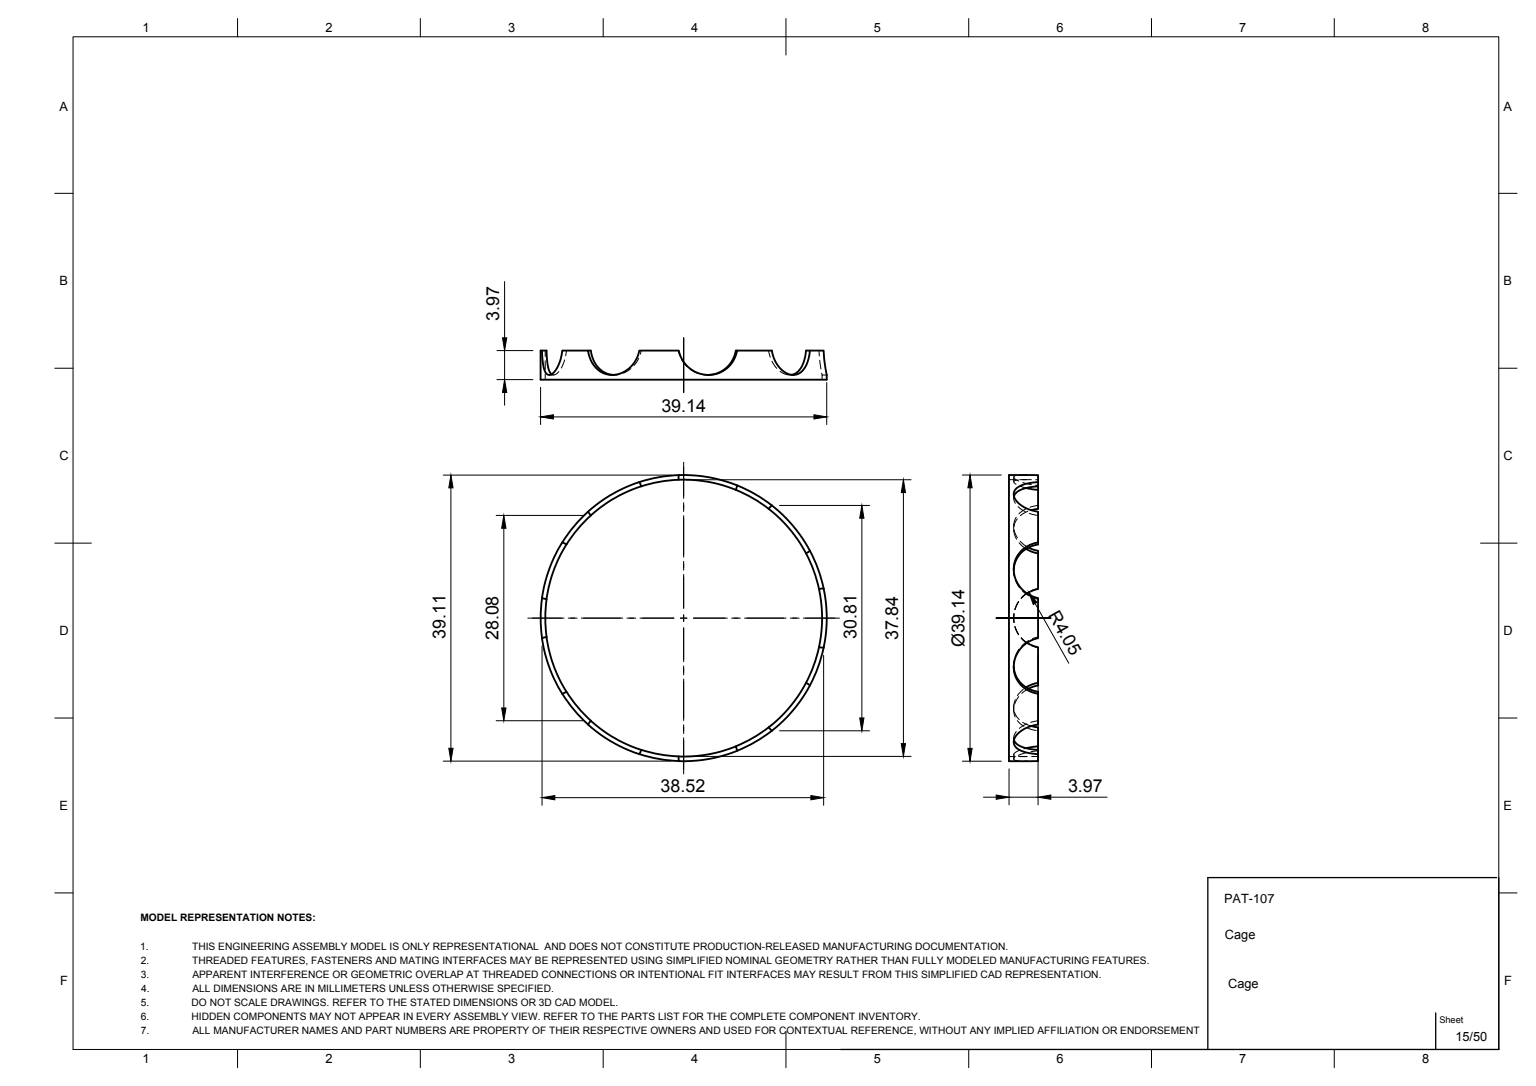
ISO-10303-21;
HEADER;
/* Generated by software containing ST-Developer
 * from STEP Tools, Inc. (www.steptools.com) 
 */

FILE_DESCRIPTION(
/* description */ ('Turntable on roller ring'),
/* implementation_level */ '2;1');

FILE_NAME(
/* name */ 'Cage.step',
/* time_stamp */ '2026-10-28T03:23:59-07:00',
/* author */ (''),
/* organization */ (''),
/* preprocessor_version */ 'ST-DEVELOPER v20.2',
/* originating_system */ 'Autodesk Translation Framework v15.17.0.0',
/* authorisation */ '');

FILE_SCHEMA (('AUTOMOTIVE_DESIGN { 1 0 10303 214 3 1 1 }'));
ENDSEC;

DATA;
#10=MECHANICAL_DESIGN_GEOMETRIC_PRESENTATION_REPRESENTATION('',(#632),#16281);
#399=B_SPLINE_CURVE_WITH_KNOTS('',3,(#13508,#13509,#13510,#13511,#13512,
#13513,#13514,#13515,#13516,#13517,#13518,#13519,#13520,#13521,#13522,#13523,
#13524,#13525,#13526,#13527,#13528,#13529),.UNSPECIFIED.,.F.,.F.,(4,2,2,
2,2,2,2,2,2,2,4),(0.0789043916784349,0.21052649634152,0.31578974451228,
0.421052992683041,0.522171766675512,0.623290540667983,0.724409314660453,
0.825528088652924,0.930791336823684,1.03605458499444,1.16767668965753),
 .UNSPECIFIED.);
#400=B_SPLINE_CURVE_WITH_KNOTS('',3,(#13533,#13534,#13535,#13536,#13537,
#13538,#13539,#13540,#13541,#13542,#13543,#13544,#13545,#13546,#13547,#13548,
#13549,#13550,#13551,#13552,#13553,#13554),.UNSPECIFIED.,.F.,.F.,(4,2,2,
2,2,2,2,2,2,2,4),(0.0774711646211702,0.142095081356994,0.284190162713987,
0.410912155766437,0.514012992401139,0.617113829035841,0.720214665670543,
0.823315502305246,0.950037495357694,1.09213257671469,1.15675649345051),
 .UNSPECIFIED.);
#401=B_SPLINE_CURVE_WITH_KNOTS('',3,(#13560,#13561,#13562,#13563,#13564,
#13565,#13566,#13567,#13568,#13569,#13570,#13571,#13572,#13573,#13574,#13575,
#13576,#13577,#13578,#13579,#13580,#13581),.UNSPECIFIED.,.F.,.F.,(4,2,2,
2,2,2,2,2,2,2,4),(0.0774711646211703,0.142095081356994,0.284190162713988,
0.410912155766436,0.514012992401139,0.617113829035841,0.720214665670544,
0.823315502305246,0.950037495357695,1.09213257671469,1.15675649345051),
 .UNSPECIFIED.);
#402=B_SPLINE_CURVE_WITH_KNOTS('',3,(#13585,#13586,#13587,#13588,#13589,
#13590,#13591,#13592,#13593,#13594,#13595,#13596,#13597,#13598,#13599,#13600,
#13601,#13602,#13603,#13604,#13605,#13606),.UNSPECIFIED.,.F.,.F.,(4,2,2,
2,2,2,2,2,2,2,4),(0.0774711646211702,0.142095081356994,0.284190162713988,
0.410912155766436,0.514012992401139,0.617113829035841,0.720214665670544,
0.823315502305246,0.950037495357695,1.09213257671469,1.15675649345051),
 .UNSPECIFIED.);
#403=B_SPLINE_CURVE_WITH_KNOTS('',3,(#13610,#13611,#13612,#13613,#13614,
#13615,#13616,#13617,#13618,#13619,#13620,#13621,#13622,#13623,#13624,#13625,
#13626,#13627,#13628,#13629,#13630,#13631),.UNSPECIFIED.,.F.,.F.,(4,2,2,
2,2,2,2,2,2,2,4),(0.0774711646211702,0.142095081356994,0.284190162713988,
0.410912155766436,0.514012992401139,0.617113829035842,0.720214665670544,
0.823315502305246,0.950037495357696,1.09213257671469,1.15675649345051),
 .UNSPECIFIED.);
#404=B_SPLINE_CURVE_WITH_KNOTS('',3,(#13640,#13641,#13642,#13643,#13644,
#13645,#13646,#13647,#13648,#13649,#13650,#13651,#13652,#13653,#13654,#13655,
#13656,#13657,#13658,#13659,#13660,#13661),.UNSPECIFIED.,.F.,.F.,(4,2,2,
2,2,2,2,2,2,2,4),(0.0774711646211702,0.142095081356994,0.284190162713987,
0.410912155766436,0.514012992401139,0.617113829035841,0.720214665670543,
0.823315502305246,0.950037495357695,1.09213257671469,1.15675649345051),
 .UNSPECIFIED.);
#405=B_SPLINE_CURVE_WITH_KNOTS('',3,(#13665,#13666,#13667,#13668,#13669,
#13670,#13671,#13672,#13673,#13674,#13675,#13676,#13677,#13678,#13679,#13680,
#13681,#13682,#13683,#13684,#13685,#13686),.UNSPECIFIED.,.F.,.F.,(4,2,2,
2,2,2,2,2,2,2,4),(0.0774711646211702,0.142095081356994,0.284190162713987,
0.410912155766436,0.514012992401139,0.617113829035841,0.720214665670543,
0.823315502305246,0.950037495357695,1.09213257671469,1.15675649345051),
 .UNSPECIFIED.);
#406=B_SPLINE_CURVE_WITH_KNOTS('',3,(#13690,#13691,#13692,#13693,#13694,
#13695,#13696,#13697,#13698,#13699,#13700,#13701,#13702,#13703,#13704,#13705,
#13706,#13707,#13708,#13709,#13710,#13711),.UNSPECIFIED.,.F.,.F.,(4,2,2,
2,2,2,2,2,2,2,4),(0.0774711646211703,0.142095081356994,0.284190162713988,
0.410912155766437,0.514012992401139,0.617113829035841,0.720214665670544,
0.823315502305247,0.950037495357696,1.09213257671469,1.15675649345051),
 .UNSPECIFIED.);
#407=B_SPLINE_CURVE_WITH_KNOTS('',3,(#13715,#13716,#13717,#13718,#13719,
#13720,#13721,#13722,#13723,#13724,#13725,#13726,#13727,#13728,#13729,#13730,
#13731,#13732,#13733,#13734,#13735,#13736),.UNSPECIFIED.,.F.,.F.,(4,2,2,
2,2,2,2,2,2,2,4),(0.0774711646211703,0.142095081356994,0.284190162713987,
0.410912155766436,0.514012992401139,0.617113829035841,0.720214665670543,
0.823315502305245,0.950037495357694,1.09213257671469,1.15675649345051),
 .UNSPECIFIED.);
#408=B_SPLINE_CURVE_WITH_KNOTS('',3,(#13740,#13741,#13742,#13743,#13744,
#13745,#13746,#13747,#13748,#13749,#13750,#13751,#13752,#13753,#13754,#13755,
#13756,#13757,#13758,#13759,#13760,#13761),.UNSPECIFIED.,.F.,.F.,(4,2,2,
2,2,2,2,2,2,2,4),(0.0774711646211703,0.142095081356994,0.284190162713988,
0.410912155766437,0.514012992401139,0.617113829035841,0.720214665670544,
0.823315502305246,0.950037495357695,1.09213257671469,1.15675649345051),
 .UNSPECIFIED.);
#409=B_SPLINE_CURVE_WITH_KNOTS('',3,(#13769,#13770,#13771,#13772,#13773,
#13774,#13775,#13776,#13777,#13778,#13779,#13780,#13781,#13782,#13783,#13784,
#13785,#13786,#13787,#13788,#13789,#13790),.UNSPECIFIED.,.F.,.F.,(4,2,2,
2,2,2,2,2,2,2,4),(0.0789043916784349,0.21052649634152,0.315789744512281,
0.421052992683041,0.522171766675512,0.623290540667983,0.724409314660453,
0.825528088652924,0.930791336823684,1.03605458499444,1.16767668965753),
 .UNSPECIFIED.);
#410=B_SPLINE_CURVE_WITH_KNOTS('',3,(#13798,#13799,#13800,#13801,#13802,
#13803,#13804,#13805,#13806,#13807,#13808,#13809,#13810,#13811,#13812,#13813,
#13814,#13815,#13816,#13817,#13818,#13819),.UNSPECIFIED.,.F.,.F.,(4,2,2,
2,2,2,2,2,2,2,4),(0.0789043916784348,0.210526496341521,0.315789744512281,
0.421052992683042,0.522171766675513,0.623290540667983,0.724409314660454,
0.825528088652925,0.930791336823685,1.03605458499444,1.16767668965753),
 .UNSPECIFIED.);
#411=B_SPLINE_CURVE_WITH_KNOTS('',3,(#13827,#13828,#13829,#13830,#13831,
#13832,#13833,#13834,#13835,#13836,#13837,#13838,#13839,#13840,#13841,#13842,
#13843,#13844,#13845,#13846,#13847,#13848),.UNSPECIFIED.,.F.,.F.,(4,2,2,
2,2,2,2,2,2,2,4),(0.0789043916784349,0.21052649634152,0.31578974451228,
0.421052992683041,0.522171766675511,0.623290540667982,0.724409314660453,
0.825528088652924,0.930791336823685,1.03605458499444,1.16767668965753),
 .UNSPECIFIED.);
#412=B_SPLINE_CURVE_WITH_KNOTS('',3,(#13858,#13859,#13860,#13861,#13862,
#13863,#13864,#13865,#13866,#13867,#13868,#13869,#13870,#13871,#13872,#13873,
#13874,#13875,#13876,#13877,#13878,#13879),.UNSPECIFIED.,.F.,.F.,(4,2,2,
2,2,2,2,2,2,2,4),(0.0789043916784348,0.21052649634152,0.315789744512281,
0.421052992683041,0.522171766675511,0.623290540667982,0.724409314660453,
0.825528088652924,0.930791336823684,1.03605458499444,1.16767668965753),
 .UNSPECIFIED.);
#413=B_SPLINE_CURVE_WITH_KNOTS('',3,(#13887,#13888,#13889,#13890,#13891,
#13892,#13893,#13894,#13895,#13896,#13897,#13898,#13899,#13900,#13901,#13902,
#13903,#13904,#13905,#13906,#13907,#13908),.UNSPECIFIED.,.F.,.F.,(4,2,2,
2,2,2,2,2,2,2,4),(0.0789043916784348,0.21052649634152,0.31578974451228,
0.42105299268304,0.522171766675511,0.623290540667982,0.724409314660453,
0.825528088652924,0.930791336823684,1.03605458499444,1.16767668965753),
 .UNSPECIFIED.);
#414=B_SPLINE_CURVE_WITH_KNOTS('',3,(#13916,#13917,#13918,#13919,#13920,
#13921,#13922,#13923,#13924,#13925,#13926,#13927,#13928,#13929,#13930,#13931,
#13932,#13933,#13934,#13935,#13936,#13937),.UNSPECIFIED.,.F.,.F.,(4,2,2,
2,2,2,2,2,2,2,4),(0.0789043916784348,0.21052649634152,0.315789744512281,
0.421052992683041,0.522171766675512,0.623290540667982,0.724409314660453,
0.825528088652924,0.930791336823684,1.03605458499444,1.16767668965753),
 .UNSPECIFIED.);
#415=B_SPLINE_CURVE_WITH_KNOTS('',3,(#13945,#13946,#13947,#13948,#13949,
#13950,#13951,#13952,#13953,#13954,#13955,#13956,#13957,#13958,#13959,#13960,
#13961,#13962,#13963,#13964,#13965,#13966),.UNSPECIFIED.,.F.,.F.,(4,2,2,
2,2,2,2,2,2,2,4),(0.0789043916784349,0.21052649634152,0.31578974451228,
0.42105299268304,0.522171766675511,0.623290540667982,0.724409314660453,
0.825528088652924,0.930791336823684,1.03605458499444,1.16767668965753),
 .UNSPECIFIED.);
#416=B_SPLINE_CURVE_WITH_KNOTS('',3,(#13975,#13976,#13977,#13978,#13979,
#13980,#13981,#13982,#13983,#13984,#13985,#13986,#13987,#13988,#13989,#13990,
#13991,#13992,#13993,#13994,#13995,#13996),.UNSPECIFIED.,.F.,.F.,(4,2,2,
2,2,2,2,2,2,2,4),(0.0789043916784348,0.21052649634152,0.31578974451228,
0.42105299268304,0.522171766675511,0.623290540667982,0.724409314660453,
0.825528088652924,0.930791336823684,1.03605458499444,1.16767668965753),
 .UNSPECIFIED.);
#447=SPHERICAL_SURFACE('',#9291,0.412776);
#448=SPHERICAL_SURFACE('',#9309,0.412776);
#449=SPHERICAL_SURFACE('',#9314,0.412776);
#450=SPHERICAL_SURFACE('',#9319,0.412776);
#451=SPHERICAL_SURFACE('',#9325,0.412776);
#452=SPHERICAL_SURFACE('',#9330,0.412776);
#453=SPHERICAL_SURFACE('',#9335,0.412776);
#454=SPHERICAL_SURFACE('',#9340,0.412776);
#455=SPHERICAL_SURFACE('',#9348,0.412776);
#514=SHAPE_REPRESENTATION_RELATIONSHIP('SRR','None',#16529,#569);
#569=ADVANCED_BREP_SHAPE_REPRESENTATION('',(#703),#16223);
#632=STYLED_ITEM('',(#16932),#703);
#703=MANIFOLD_SOLID_BREP('Continuous crown cage',#8374);
#828=FACE_BOUND('',#1953,.T.);
#1025=PLANE('',#9306);
#1026=PLANE('',#9311);
#1027=PLANE('',#9316);
#1028=PLANE('',#9321);
#1029=PLANE('',#9327);
#1030=PLANE('',#9332);
#1031=PLANE('',#9337);
#1032=PLANE('',#9346);
#1033=PLANE('',#9350);
#1034=PLANE('',#9351);
#1357=FACE_OUTER_BOUND('',#1933,.T.);
#1358=FACE_OUTER_BOUND('',#1934,.T.);
#1359=FACE_OUTER_BOUND('',#1935,.T.);
#1360=FACE_OUTER_BOUND('',#1936,.T.);
#1361=FACE_OUTER_BOUND('',#1937,.T.);
#1362=FACE_OUTER_BOUND('',#1938,.T.);
#1363=FACE_OUTER_BOUND('',#1939,.T.);
#1364=FACE_OUTER_BOUND('',#1940,.T.);
#1365=FACE_OUTER_BOUND('',#1941,.T.);
#1366=FACE_OUTER_BOUND('',#1942,.T.);
#1367=FACE_OUTER_BOUND('',#1943,.T.);
#1368=FACE_OUTER_BOUND('',#1944,.T.);
#1369=FACE_OUTER_BOUND('',#1945,.T.);
#1370=FACE_OUTER_BOUND('',#1946,.T.);
#1371=FACE_OUTER_BOUND('',#1947,.T.);
#1372=FACE_OUTER_BOUND('',#1948,.T.);
#1373=FACE_OUTER_BOUND('',#1949,.T.);
#1374=FACE_OUTER_BOUND('',#1950,.T.);
#1375=FACE_OUTER_BOUND('',#1951,.T.);
#1376=FACE_OUTER_BOUND('',#1952,.T.);
#1377=FACE_OUTER_BOUND('',#1954,.T.);
#1933=EDGE_LOOP('',(#6101,#6102,#6103,#6104));
#1934=EDGE_LOOP('',(#6105,#6106,#6107,#6108,#6109,#6110,#6111,#6112,#6113,
#6114,#6115,#6116,#6117,#6118,#6119,#6120,#6121,#6122,#6123,#6124,#6125,
#6126));
#1935=EDGE_LOOP('',(#6127,#6128,#6129,#6130));
#1936=EDGE_LOOP('',(#6131,#6132,#6133,#6134));
#1937=EDGE_LOOP('',(#6135,#6136,#6137,#6138));
#1938=EDGE_LOOP('',(#6139,#6140,#6141,#6142));
#1939=EDGE_LOOP('',(#6143,#6144,#6145,#6146));
#1940=EDGE_LOOP('',(#6147,#6148,#6149,#6150));
#1941=EDGE_LOOP('',(#6151,#6152,#6153,#6154,#6155,#6156));
#1942=EDGE_LOOP('',(#6157,#6158,#6159,#6160));
#1943=EDGE_LOOP('',(#6161,#6162,#6163,#6164));
#1944=EDGE_LOOP('',(#6165,#6166,#6167,#6168));
#1945=EDGE_LOOP('',(#6169,#6170,#6171,#6172));
#1946=EDGE_LOOP('',(#6173,#6174,#6175,#6176));
#1947=EDGE_LOOP('',(#6177,#6178,#6179,#6180));
#1948=EDGE_LOOP('',(#6181,#6182,#6183,#6184));
#1949=EDGE_LOOP('',(#6185,#6186,#6187,#6188,#6189,#6190,#6191,#6192,#6193,
#6194,#6195,#6196,#6197,#6198,#6199,#6200,#6201,#6202,#6203,#6204,#6205,
#6206));
#1950=EDGE_LOOP('',(#6207,#6208,#6209,#6210));
#1951=EDGE_LOOP('',(#6211,#6212,#6213,#6214));
#1952=EDGE_LOOP('',(#6215));
#1953=EDGE_LOOP('',(#6216));
#1954=EDGE_LOOP('',(#6217,#6218,#6219,#6220));
#2588=LINE('',#13635,#3071);
#2589=LINE('',#13971,#3072);
#3071=VECTOR('',#10813,1.956752);
#3072=VECTOR('',#10904,1.893248);
#3592=CIRCLE('',#9292,0.405071403305639);
#3593=CIRCLE('',#9293,0.405071403305639);
#3594=CIRCLE('',#9295,1.956752);
#3595=CIRCLE('',#9296,1.956752);
#3596=CIRCLE('',#9297,1.956752);
#3597=CIRCLE('',#9298,1.956752);
#3598=CIRCLE('',#9299,1.956752);
#3599=CIRCLE('',#9300,1.956752);
#3600=CIRCLE('',#9301,1.956752);
#3601=CIRCLE('',#9302,1.956752);
#3602=CIRCLE('',#9303,1.956752);
#3603=CIRCLE('',#9304,1.956752);
#3604=CIRCLE('',#9305,1.956752);
#3605=CIRCLE('',#9307,1.893248);
#3606=CIRCLE('',#9308,0.405071403305639);
#3607=CIRCLE('',#9310,0.405071403305639);
#3608=CIRCLE('',#9312,1.893248);
#3609=CIRCLE('',#9313,0.405071403305639);
#3610=CIRCLE('',#9315,0.405071403305639);
#3611=CIRCLE('',#9317,1.893248);
#3612=CIRCLE('',#9318,0.405071403305639);
#3613=CIRCLE('',#9320,0.405071403305639);
#3614=CIRCLE('',#9322,1.893248);
#3615=CIRCLE('',#9323,1.893248);
#3616=CIRCLE('',#9324,0.405071403305639);
#3617=CIRCLE('',#9326,0.405071403305639);
#3618=CIRCLE('',#9328,1.893248);
#3619=CIRCLE('',#9329,0.405071403305639);
#3620=CIRCLE('',#9331,0.405071403305639);
#3621=CIRCLE('',#9333,1.893248);
#3622=CIRCLE('',#9334,0.405071403305639);
#3623=CIRCLE('',#9336,0.405071403305639);
#3624=CIRCLE('',#9338,1.893248);
#3625=CIRCLE('',#9339,0.405071403305639);
#3626=CIRCLE('',#9341,0.405071403305639);
#3627=CIRCLE('',#9343,1.893248);
#3628=CIRCLE('',#9344,1.893248);
#3629=CIRCLE('',#9345,1.893248);
#3630=CIRCLE('',#9347,0.405071403305639);
#3631=CIRCLE('',#9349,0.405071403305639);
#4105=VERTEX_POINT('',#13506);
#4106=VERTEX_POINT('',#13507);
#4107=VERTEX_POINT('',#13530);
#4108=VERTEX_POINT('',#13532);
#4109=VERTEX_POINT('',#13557);
#4110=VERTEX_POINT('',#13559);
#4111=VERTEX_POINT('',#13582);
#4112=VERTEX_POINT('',#13584);
#4113=VERTEX_POINT('',#13607);
#4114=VERTEX_POINT('',#13609);
#4115=VERTEX_POINT('',#13632);
#4116=VERTEX_POINT('',#13634);
#4117=VERTEX_POINT('',#13637);
#4118=VERTEX_POINT('',#13639);
#4119=VERTEX_POINT('',#13662);
#4120=VERTEX_POINT('',#13664);
#4121=VERTEX_POINT('',#13687);
#4122=VERTEX_POINT('',#13689);
#4123=VERTEX_POINT('',#13712);
#4124=VERTEX_POINT('',#13714);
#4125=VERTEX_POINT('',#13737);
#4126=VERTEX_POINT('',#13739);
#4127=VERTEX_POINT('',#13764);
#4128=VERTEX_POINT('',#13768);
#4129=VERTEX_POINT('',#13793);
#4130=VERTEX_POINT('',#13797);
#4131=VERTEX_POINT('',#13822);
#4132=VERTEX_POINT('',#13826);
#4133=VERTEX_POINT('',#13851);
#4134=VERTEX_POINT('',#13853);
#4135=VERTEX_POINT('',#13857);
#4136=VERTEX_POINT('',#13882);
#4137=VERTEX_POINT('',#13886);
#4138=VERTEX_POINT('',#13911);
#4139=VERTEX_POINT('',#13915);
#4140=VERTEX_POINT('',#13940);
#4141=VERTEX_POINT('',#13944);
#4142=VERTEX_POINT('',#13969);
#4143=VERTEX_POINT('',#13972);
#4144=VERTEX_POINT('',#13974);
#4861=EDGE_CURVE('',#4105,#4106,#399,.T.);
#4862=EDGE_CURVE('',#4107,#4105,#3592,.T.);
#4863=EDGE_CURVE('',#4108,#4107,#400,.T.);
#4864=EDGE_CURVE('',#4106,#4108,#3593,.T.);
#4865=EDGE_CURVE('',#4109,#4107,#3594,.T.);
#4866=EDGE_CURVE('',#4109,#4110,#401,.T.);
#4867=EDGE_CURVE('',#4111,#4110,#3595,.T.);
#4868=EDGE_CURVE('',#4111,#4112,#402,.T.);
#4869=EDGE_CURVE('',#4113,#4112,#3596,.T.);
#4870=EDGE_CURVE('',#4113,#4114,#403,.T.);
#4871=EDGE_CURVE('',#4115,#4114,#3597,.T.);
#4872=EDGE_CURVE('',#4115,#4116,#2588,.T.);
#4873=EDGE_CURVE('',#4116,#4116,#3598,.T.);
#4874=EDGE_CURVE('',#4117,#4115,#3599,.T.);
#4875=EDGE_CURVE('',#4117,#4118,#404,.T.);
#4876=EDGE_CURVE('',#4119,#4118,#3600,.T.);
#4877=EDGE_CURVE('',#4119,#4120,#405,.T.);
#4878=EDGE_CURVE('',#4121,#4120,#3601,.T.);
#4879=EDGE_CURVE('',#4121,#4122,#406,.T.);
#4880=EDGE_CURVE('',#4123,#4122,#3602,.T.);
#4881=EDGE_CURVE('',#4123,#4124,#407,.T.);
#4882=EDGE_CURVE('',#4125,#4124,#3603,.T.);
#4883=EDGE_CURVE('',#4125,#4126,#408,.T.);
#4884=EDGE_CURVE('',#4108,#4126,#3604,.T.);
#4885=EDGE_CURVE('',#4105,#4127,#3605,.T.);
#4886=EDGE_CURVE('',#4127,#4109,#3606,.T.);
#4887=EDGE_CURVE('',#4128,#4127,#409,.T.);
#4888=EDGE_CURVE('',#4110,#4128,#3607,.T.);
#4889=EDGE_CURVE('',#4128,#4129,#3608,.T.);
#4890=EDGE_CURVE('',#4129,#4111,#3609,.T.);
#4891=EDGE_CURVE('',#4130,#4129,#410,.T.);
#4892=EDGE_CURVE('',#4112,#4130,#3610,.T.);
#4893=EDGE_CURVE('',#4130,#4131,#3611,.T.);
#4894=EDGE_CURVE('',#4131,#4113,#3612,.T.);
#4895=EDGE_CURVE('',#4132,#4131,#411,.T.);
#4896=EDGE_CURVE('',#4114,#4132,#3613,.T.);
#4897=EDGE_CURVE('',#4132,#4133,#3614,.T.);
#4898=EDGE_CURVE('',#4133,#4134,#3615,.T.);
#4899=EDGE_CURVE('',#4134,#4117,#3616,.T.);
#4900=EDGE_CURVE('',#4135,#4134,#412,.T.);
#4901=EDGE_CURVE('',#4118,#4135,#3617,.T.);
#4902=EDGE_CURVE('',#4135,#4136,#3618,.T.);
#4903=EDGE_CURVE('',#4136,#4119,#3619,.T.);
#4904=EDGE_CURVE('',#4137,#4136,#413,.T.);
#4905=EDGE_CURVE('',#4120,#4137,#3620,.T.);
#4906=EDGE_CURVE('',#4137,#4138,#3621,.T.);
#4907=EDGE_CURVE('',#4138,#4121,#3622,.T.);
#4908=EDGE_CURVE('',#4139,#4138,#414,.T.);
#4909=EDGE_CURVE('',#4122,#4139,#3623,.T.);
#4910=EDGE_CURVE('',#4139,#4140,#3624,.T.);
#4911=EDGE_CURVE('',#4140,#4123,#3625,.T.);
#4912=EDGE_CURVE('',#4141,#4140,#415,.T.);
#4913=EDGE_CURVE('',#4124,#4141,#3626,.T.);
#4914=EDGE_CURVE('',#4142,#4142,#3627,.T.);
#4915=EDGE_CURVE('',#4142,#4133,#2589,.T.);
#4916=EDGE_CURVE('',#4143,#4106,#3628,.T.);
#4917=EDGE_CURVE('',#4143,#4144,#416,.T.);
#4918=EDGE_CURVE('',#4141,#4144,#3629,.T.);
#4919=EDGE_CURVE('',#4126,#4143,#3630,.T.);
#4920=EDGE_CURVE('',#4144,#4125,#3631,.T.);
#6101=ORIENTED_EDGE('',*,*,#4861,.F.);
#6102=ORIENTED_EDGE('',*,*,#4862,.F.);
#6103=ORIENTED_EDGE('',*,*,#4863,.F.);
#6104=ORIENTED_EDGE('',*,*,#4864,.F.);
#6105=ORIENTED_EDGE('',*,*,#4863,.T.);
#6106=ORIENTED_EDGE('',*,*,#4865,.F.);
#6107=ORIENTED_EDGE('',*,*,#4866,.T.);
#6108=ORIENTED_EDGE('',*,*,#4867,.F.);
#6109=ORIENTED_EDGE('',*,*,#4868,.T.);
#6110=ORIENTED_EDGE('',*,*,#4869,.F.);
#6111=ORIENTED_EDGE('',*,*,#4870,.T.);
#6112=ORIENTED_EDGE('',*,*,#4871,.F.);
#6113=ORIENTED_EDGE('',*,*,#4872,.T.);
#6114=ORIENTED_EDGE('',*,*,#4873,.F.);
#6115=ORIENTED_EDGE('',*,*,#4872,.F.);
#6116=ORIENTED_EDGE('',*,*,#4874,.F.);
#6117=ORIENTED_EDGE('',*,*,#4875,.T.);
#6118=ORIENTED_EDGE('',*,*,#4876,.F.);
#6119=ORIENTED_EDGE('',*,*,#4877,.T.);
#6120=ORIENTED_EDGE('',*,*,#4878,.F.);
#6121=ORIENTED_EDGE('',*,*,#4879,.T.);
#6122=ORIENTED_EDGE('',*,*,#4880,.F.);
#6123=ORIENTED_EDGE('',*,*,#4881,.T.);
#6124=ORIENTED_EDGE('',*,*,#4882,.F.);
#6125=ORIENTED_EDGE('',*,*,#4883,.T.);
#6126=ORIENTED_EDGE('',*,*,#4884,.F.);
#6127=ORIENTED_EDGE('',*,*,#4862,.T.);
#6128=ORIENTED_EDGE('',*,*,#4885,.T.);
#6129=ORIENTED_EDGE('',*,*,#4886,.T.);
#6130=ORIENTED_EDGE('',*,*,#4865,.T.);
#6131=ORIENTED_EDGE('',*,*,#4887,.F.);
#6132=ORIENTED_EDGE('',*,*,#4888,.F.);
#6133=ORIENTED_EDGE('',*,*,#4866,.F.);
#6134=ORIENTED_EDGE('',*,*,#4886,.F.);
#6135=ORIENTED_EDGE('',*,*,#4888,.T.);
#6136=ORIENTED_EDGE('',*,*,#4889,.T.);
#6137=ORIENTED_EDGE('',*,*,#4890,.T.);
#6138=ORIENTED_EDGE('',*,*,#4867,.T.);
#6139=ORIENTED_EDGE('',*,*,#4891,.F.);
#6140=ORIENTED_EDGE('',*,*,#4892,.F.);
#6141=ORIENTED_EDGE('',*,*,#4868,.F.);
#6142=ORIENTED_EDGE('',*,*,#4890,.F.);
#6143=ORIENTED_EDGE('',*,*,#4892,.T.);
#6144=ORIENTED_EDGE('',*,*,#4893,.T.);
#6145=ORIENTED_EDGE('',*,*,#4894,.T.);
#6146=ORIENTED_EDGE('',*,*,#4869,.T.);
#6147=ORIENTED_EDGE('',*,*,#4895,.F.);
#6148=ORIENTED_EDGE('',*,*,#4896,.F.);
#6149=ORIENTED_EDGE('',*,*,#4870,.F.);
#6150=ORIENTED_EDGE('',*,*,#4894,.F.);
#6151=ORIENTED_EDGE('',*,*,#4896,.T.);
#6152=ORIENTED_EDGE('',*,*,#4897,.T.);
#6153=ORIENTED_EDGE('',*,*,#4898,.T.);
#6154=ORIENTED_EDGE('',*,*,#4899,.T.);
#6155=ORIENTED_EDGE('',*,*,#4874,.T.);
#6156=ORIENTED_EDGE('',*,*,#4871,.T.);
#6157=ORIENTED_EDGE('',*,*,#4900,.F.);
#6158=ORIENTED_EDGE('',*,*,#4901,.F.);
#6159=ORIENTED_EDGE('',*,*,#4875,.F.);
#6160=ORIENTED_EDGE('',*,*,#4899,.F.);
#6161=ORIENTED_EDGE('',*,*,#4901,.T.);
#6162=ORIENTED_EDGE('',*,*,#4902,.T.);
#6163=ORIENTED_EDGE('',*,*,#4903,.T.);
#6164=ORIENTED_EDGE('',*,*,#4876,.T.);
#6165=ORIENTED_EDGE('',*,*,#4904,.F.);
#6166=ORIENTED_EDGE('',*,*,#4905,.F.);
#6167=ORIENTED_EDGE('',*,*,#4877,.F.);
#6168=ORIENTED_EDGE('',*,*,#4903,.F.);
#6169=ORIENTED_EDGE('',*,*,#4905,.T.);
#6170=ORIENTED_EDGE('',*,*,#4906,.T.);
#6171=ORIENTED_EDGE('',*,*,#4907,.T.);
#6172=ORIENTED_EDGE('',*,*,#4878,.T.);
#6173=ORIENTED_EDGE('',*,*,#4908,.F.);
#6174=ORIENTED_EDGE('',*,*,#4909,.F.);
#6175=ORIENTED_EDGE('',*,*,#4879,.F.);
#6176=ORIENTED_EDGE('',*,*,#4907,.F.);
#6177=ORIENTED_EDGE('',*,*,#4909,.T.);
#6178=ORIENTED_EDGE('',*,*,#4910,.T.);
#6179=ORIENTED_EDGE('',*,*,#4911,.T.);
#6180=ORIENTED_EDGE('',*,*,#4880,.T.);
#6181=ORIENTED_EDGE('',*,*,#4881,.F.);
#6182=ORIENTED_EDGE('',*,*,#4911,.F.);
#6183=ORIENTED_EDGE('',*,*,#4912,.F.);
#6184=ORIENTED_EDGE('',*,*,#4913,.F.);
#6185=ORIENTED_EDGE('',*,*,#4914,.F.);
#6186=ORIENTED_EDGE('',*,*,#4915,.T.);
#6187=ORIENTED_EDGE('',*,*,#4897,.F.);
#6188=ORIENTED_EDGE('',*,*,#4895,.T.);
#6189=ORIENTED_EDGE('',*,*,#4893,.F.);
#6190=ORIENTED_EDGE('',*,*,#4891,.T.);
#6191=ORIENTED_EDGE('',*,*,#4889,.F.);
#6192=ORIENTED_EDGE('',*,*,#4887,.T.);
#6193=ORIENTED_EDGE('',*,*,#4885,.F.);
#6194=ORIENTED_EDGE('',*,*,#4861,.T.);
#6195=ORIENTED_EDGE('',*,*,#4916,.F.);
#6196=ORIENTED_EDGE('',*,*,#4917,.T.);
#6197=ORIENTED_EDGE('',*,*,#4918,.F.);
#6198=ORIENTED_EDGE('',*,*,#4912,.T.);
#6199=ORIENTED_EDGE('',*,*,#4910,.F.);
#6200=ORIENTED_EDGE('',*,*,#4908,.T.);
#6201=ORIENTED_EDGE('',*,*,#4906,.F.);
#6202=ORIENTED_EDGE('',*,*,#4904,.T.);
#6203=ORIENTED_EDGE('',*,*,#4902,.F.);
#6204=ORIENTED_EDGE('',*,*,#4900,.T.);
#6205=ORIENTED_EDGE('',*,*,#4898,.F.);
#6206=ORIENTED_EDGE('',*,*,#4915,.F.);
#6207=ORIENTED_EDGE('',*,*,#4864,.T.);
#6208=ORIENTED_EDGE('',*,*,#4884,.T.);
#6209=ORIENTED_EDGE('',*,*,#4919,.T.);
#6210=ORIENTED_EDGE('',*,*,#4916,.T.);
#6211=ORIENTED_EDGE('',*,*,#4883,.F.);
#6212=ORIENTED_EDGE('',*,*,#4920,.F.);
#6213=ORIENTED_EDGE('',*,*,#4917,.F.);
#6214=ORIENTED_EDGE('',*,*,#4919,.F.);
#6215=ORIENTED_EDGE('',*,*,#4873,.T.);
#6216=ORIENTED_EDGE('',*,*,#4914,.T.);
#6217=ORIENTED_EDGE('',*,*,#4913,.T.);
#6218=ORIENTED_EDGE('',*,*,#4918,.T.);
#6219=ORIENTED_EDGE('',*,*,#4920,.T.);
#6220=ORIENTED_EDGE('',*,*,#4882,.T.);
#7723=CYLINDRICAL_SURFACE('',#9294,1.956752);
#7724=CYLINDRICAL_SURFACE('',#9342,1.893248);
#7960=ADVANCED_FACE('',(#1357),#447,.F.);
#7961=ADVANCED_FACE('',(#1358),#7723,.T.);
#7962=ADVANCED_FACE('',(#1359),#1025,.T.);
#7963=ADVANCED_FACE('',(#1360),#448,.F.);
#7964=ADVANCED_FACE('',(#1361),#1026,.T.);
#7965=ADVANCED_FACE('',(#1362),#449,.F.);
#7966=ADVANCED_FACE('',(#1363),#1027,.T.);
#7967=ADVANCED_FACE('',(#1364),#450,.F.);
#7968=ADVANCED_FACE('',(#1365),#1028,.T.);
#7969=ADVANCED_FACE('',(#1366),#451,.F.);
#7970=ADVANCED_FACE('',(#1367),#1029,.T.);
#7971=ADVANCED_FACE('',(#1368),#452,.F.);
#7972=ADVANCED_FACE('',(#1369),#1030,.T.);
#7973=ADVANCED_FACE('',(#1370),#453,.F.);
#7974=ADVANCED_FACE('',(#1371),#1031,.T.);
#7975=ADVANCED_FACE('',(#1372),#454,.F.);
#7976=ADVANCED_FACE('',(#1373),#7724,.F.);
#7977=ADVANCED_FACE('',(#1374),#1032,.T.);
#7978=ADVANCED_FACE('',(#1375),#455,.F.);
#7979=ADVANCED_FACE('',(#1376,#828),#1033,.T.);
#7980=ADVANCED_FACE('',(#1377),#1034,.T.);
#8374=CLOSED_SHELL('',(#7960,#7961,#7962,#7963,#7964,#7965,#7966,#7967,
#7968,#7969,#7970,#7971,#7972,#7973,#7974,#7975,#7976,#7977,#7978,#7979,
#7980));
#9290=AXIS2_PLACEMENT_3D('',#13504,#10795,#10796);
#9291=AXIS2_PLACEMENT_3D('',#13505,#10797,#10798);
#9292=AXIS2_PLACEMENT_3D('',#13531,#10799,#10800);
#9293=AXIS2_PLACEMENT_3D('',#13555,#10801,#10802);
#9294=AXIS2_PLACEMENT_3D('',#13556,#10803,#10804);
#9295=AXIS2_PLACEMENT_3D('',#13558,#10805,#10806);
#9296=AXIS2_PLACEMENT_3D('',#13583,#10807,#10808);
#9297=AXIS2_PLACEMENT_3D('',#13608,#10809,#10810);
#9298=AXIS2_PLACEMENT_3D('',#13633,#10811,#10812);
#9299=AXIS2_PLACEMENT_3D('',#13636,#10814,#10815);
#9300=AXIS2_PLACEMENT_3D('',#13638,#10816,#10817);
#9301=AXIS2_PLACEMENT_3D('',#13663,#10818,#10819);
#9302=AXIS2_PLACEMENT_3D('',#13688,#10820,#10821);
#9303=AXIS2_PLACEMENT_3D('',#13713,#10822,#10823);
#9304=AXIS2_PLACEMENT_3D('',#13738,#10824,#10825);
#9305=AXIS2_PLACEMENT_3D('',#13762,#10826,#10827);
#9306=AXIS2_PLACEMENT_3D('',#13763,#10828,#10829);
#9307=AXIS2_PLACEMENT_3D('',#13765,#10830,#10831);
#9308=AXIS2_PLACEMENT_3D('',#13766,#10832,#10833);
#9309=AXIS2_PLACEMENT_3D('',#13767,#10834,#10835);
#9310=AXIS2_PLACEMENT_3D('',#13791,#10836,#10837);
#9311=AXIS2_PLACEMENT_3D('',#13792,#10838,#10839);
#9312=AXIS2_PLACEMENT_3D('',#13794,#10840,#10841);
#9313=AXIS2_PLACEMENT_3D('',#13795,#10842,#10843);
#9314=AXIS2_PLACEMENT_3D('',#13796,#10844,#10845);
#9315=AXIS2_PLACEMENT_3D('',#13820,#10846,#10847);
#9316=AXIS2_PLACEMENT_3D('',#13821,#10848,#10849);
#9317=AXIS2_PLACEMENT_3D('',#13823,#10850,#10851);
#9318=AXIS2_PLACEMENT_3D('',#13824,#10852,#10853);
#9319=AXIS2_PLACEMENT_3D('',#13825,#10854,#10855);
#9320=AXIS2_PLACEMENT_3D('',#13849,#10856,#10857);
#9321=AXIS2_PLACEMENT_3D('',#13850,#10858,#10859);
#9322=AXIS2_PLACEMENT_3D('',#13852,#10860,#10861);
#9323=AXIS2_PLACEMENT_3D('',#13854,#10862,#10863);
#9324=AXIS2_PLACEMENT_3D('',#13855,#10864,#10865);
#9325=AXIS2_PLACEMENT_3D('',#13856,#10866,#10867);
#9326=AXIS2_PLACEMENT_3D('',#13880,#10868,#10869);
#9327=AXIS2_PLACEMENT_3D('',#13881,#10870,#10871);
#9328=AXIS2_PLACEMENT_3D('',#13883,#10872,#10873);
#9329=AXIS2_PLACEMENT_3D('',#13884,#10874,#10875);
#9330=AXIS2_PLACEMENT_3D('',#13885,#10876,#10877);
#9331=AXIS2_PLACEMENT_3D('',#13909,#10878,#10879);
#9332=AXIS2_PLACEMENT_3D('',#13910,#10880,#10881);
#9333=AXIS2_PLACEMENT_3D('',#13912,#10882,#10883);
#9334=AXIS2_PLACEMENT_3D('',#13913,#10884,#10885);
#9335=AXIS2_PLACEMENT_3D('',#13914,#10886,#10887);
#9336=AXIS2_PLACEMENT_3D('',#13938,#10888,#10889);
#9337=AXIS2_PLACEMENT_3D('',#13939,#10890,#10891);
#9338=AXIS2_PLACEMENT_3D('',#13941,#10892,#10893);
#9339=AXIS2_PLACEMENT_3D('',#13942,#10894,#10895);
#9340=AXIS2_PLACEMENT_3D('',#13943,#10896,#10897);
#9341=AXIS2_PLACEMENT_3D('',#13967,#10898,#10899);
#9342=AXIS2_PLACEMENT_3D('',#13968,#10900,#10901);
#9343=AXIS2_PLACEMENT_3D('',#13970,#10902,#10903);
#9344=AXIS2_PLACEMENT_3D('',#13973,#10905,#10906);
#9345=AXIS2_PLACEMENT_3D('',#13997,#10907,#10908);
#9346=AXIS2_PLACEMENT_3D('',#13998,#10909,#10910);
#9347=AXIS2_PLACEMENT_3D('',#13999,#10911,#10912);
#9348=AXIS2_PLACEMENT_3D('',#14000,#10913,#10914);
#9349=AXIS2_PLACEMENT_3D('',#14001,#10915,#10916);
#9350=AXIS2_PLACEMENT_3D('',#14002,#10917,#10918);
#9351=AXIS2_PLACEMENT_3D('',#14003,#10919,#10920);
#10795=DIRECTION('axis',(0.,0.,1.));
#10796=DIRECTION('refdir',(1.,0.,0.));
#10797=DIRECTION('center_axis',(0.,0.,1.));
#10798=DIRECTION('ref_axis',(1.,0.,0.));
#10799=DIRECTION('center_axis',(0.,-1.,0.));
#10800=DIRECTION('ref_axis',(0.,0.,-1.));
#10801=DIRECTION('center_axis',(0.,-1.,0.));
#10802=DIRECTION('ref_axis',(0.,0.,-1.));
#10803=DIRECTION('center_axis',(0.,1.,0.));
#10804=DIRECTION('ref_axis',(1.,0.,0.));
#10805=DIRECTION('center_axis',(0.,1.,0.));
#10806=DIRECTION('ref_axis',(1.,0.,0.));
#10807=DIRECTION('center_axis',(0.,1.,0.));
#10808=DIRECTION('ref_axis',(1.,0.,0.));
#10809=DIRECTION('center_axis',(0.,1.,0.));
#10810=DIRECTION('ref_axis',(1.,0.,0.));
#10811=DIRECTION('center_axis',(0.,1.,0.));
#10812=DIRECTION('ref_axis',(1.,0.,0.));
#10813=DIRECTION('',(0.,-1.,0.));
#10814=DIRECTION('center_axis',(0.,-1.,0.));
#10815=DIRECTION('ref_axis',(1.,0.,0.));
#10816=DIRECTION('center_axis',(0.,1.,0.));
#10817=DIRECTION('ref_axis',(1.,0.,0.));
#10818=DIRECTION('center_axis',(0.,1.,0.));
#10819=DIRECTION('ref_axis',(1.,0.,0.));
#10820=DIRECTION('center_axis',(0.,1.,0.));
#10821=DIRECTION('ref_axis',(1.,0.,0.));
#10822=DIRECTION('center_axis',(0.,1.,0.));
#10823=DIRECTION('ref_axis',(1.,0.,0.));
#10824=DIRECTION('center_axis',(0.,1.,0.));
#10825=DIRECTION('ref_axis',(1.,0.,0.));
#10826=DIRECTION('center_axis',(0.,1.,0.));
#10827=DIRECTION('ref_axis',(1.,0.,0.));
#10828=DIRECTION('center_axis',(0.,1.,0.));
#10829=DIRECTION('ref_axis',(1.,0.,0.));
#10830=DIRECTION('center_axis',(0.,-1.,0.));
#10831=DIRECTION('ref_axis',(1.,0.,0.));
#10832=DIRECTION('center_axis',(0.,-1.,0.));
#10833=DIRECTION('ref_axis',(0.,0.,-1.));
#10834=DIRECTION('center_axis',(0.,0.,1.));
#10835=DIRECTION('ref_axis',(1.,0.,0.));
#10836=DIRECTION('center_axis',(0.,-1.,0.));
#10837=DIRECTION('ref_axis',(0.,0.,-1.));
#10838=DIRECTION('center_axis',(0.,1.,0.));
#10839=DIRECTION('ref_axis',(1.,0.,0.));
#10840=DIRECTION('center_axis',(0.,-1.,0.));
#10841=DIRECTION('ref_axis',(1.,0.,0.));
#10842=DIRECTION('center_axis',(0.,-1.,0.));
#10843=DIRECTION('ref_axis',(0.,0.,-1.));
#10844=DIRECTION('center_axis',(0.,0.,1.));
#10845=DIRECTION('ref_axis',(1.,0.,0.));
#10846=DIRECTION('center_axis',(0.,-1.,0.));
#10847=DIRECTION('ref_axis',(0.,0.,-1.));
#10848=DIRECTION('center_axis',(0.,1.,0.));
#10849=DIRECTION('ref_axis',(1.,0.,0.));
#10850=DIRECTION('center_axis',(0.,-1.,0.));
#10851=DIRECTION('ref_axis',(1.,0.,0.));
#10852=DIRECTION('center_axis',(0.,-1.,0.));
#10853=DIRECTION('ref_axis',(0.,0.,-1.));
#10854=DIRECTION('center_axis',(0.,0.,1.));
#10855=DIRECTION('ref_axis',(1.,0.,0.));
#10856=DIRECTION('center_axis',(0.,-1.,0.));
#10857=DIRECTION('ref_axis',(0.,0.,-1.));
#10858=DIRECTION('center_axis',(0.,1.,0.));
#10859=DIRECTION('ref_axis',(1.,0.,0.));
#10860=DIRECTION('center_axis',(0.,-1.,0.));
#10861=DIRECTION('ref_axis',(1.,0.,0.));
#10862=DIRECTION('center_axis',(0.,-1.,0.));
#10863=DIRECTION('ref_axis',(1.,0.,0.));
#10864=DIRECTION('center_axis',(0.,-1.,0.));
#10865=DIRECTION('ref_axis',(0.,0.,-1.));
#10866=DIRECTION('center_axis',(0.,0.,1.));
#10867=DIRECTION('ref_axis',(1.,0.,0.));
#10868=DIRECTION('center_axis',(0.,-1.,0.));
#10869=DIRECTION('ref_axis',(0.,0.,-1.));
#10870=DIRECTION('center_axis',(0.,1.,0.));
#10871=DIRECTION('ref_axis',(1.,0.,0.));
#10872=DIRECTION('center_axis',(0.,-1.,0.));
#10873=DIRECTION('ref_axis',(1.,0.,0.));
#10874=DIRECTION('center_axis',(0.,-1.,0.));
#10875=DIRECTION('ref_axis',(0.,0.,-1.));
#10876=DIRECTION('center_axis',(0.,0.,1.));
#10877=DIRECTION('ref_axis',(1.,0.,0.));
#10878=DIRECTION('center_axis',(0.,-1.,0.));
#10879=DIRECTION('ref_axis',(0.,0.,-1.));
#10880=DIRECTION('center_axis',(0.,1.,0.));
#10881=DIRECTION('ref_axis',(1.,0.,0.));
#10882=DIRECTION('center_axis',(0.,-1.,0.));
#10883=DIRECTION('ref_axis',(1.,0.,0.));
#10884=DIRECTION('center_axis',(0.,-1.,0.));
#10885=DIRECTION('ref_axis',(0.,0.,-1.));
#10886=DIRECTION('center_axis',(0.,0.,1.));
#10887=DIRECTION('ref_axis',(1.,0.,0.));
#10888=DIRECTION('center_axis',(0.,-1.,0.));
#10889=DIRECTION('ref_axis',(0.,0.,-1.));
#10890=DIRECTION('center_axis',(0.,1.,0.));
#10891=DIRECTION('ref_axis',(1.,0.,0.));
#10892=DIRECTION('center_axis',(0.,-1.,0.));
#10893=DIRECTION('ref_axis',(1.,0.,0.));
#10894=DIRECTION('center_axis',(0.,-1.,0.));
#10895=DIRECTION('ref_axis',(0.,0.,-1.));
#10896=DIRECTION('center_axis',(0.,0.,1.));
#10897=DIRECTION('ref_axis',(1.,0.,0.));
#10898=DIRECTION('center_axis',(0.,-1.,0.));
#10899=DIRECTION('ref_axis',(0.,0.,-1.));
#10900=DIRECTION('center_axis',(0.,1.,0.));
#10901=DIRECTION('ref_axis',(1.,0.,0.));
#10902=DIRECTION('center_axis',(0.,1.,0.));
#10903=DIRECTION('ref_axis',(1.,0.,0.));
#10904=DIRECTION('',(0.,1.,0.));
#10905=DIRECTION('center_axis',(0.,-1.,0.));
#10906=DIRECTION('ref_axis',(1.,0.,0.));
#10907=DIRECTION('center_axis',(0.,-1.,0.));
#10908=DIRECTION('ref_axis',(1.,0.,0.));
#10909=DIRECTION('center_axis',(0.,1.,0.));
#10910=DIRECTION('ref_axis',(1.,0.,0.));
#10911=DIRECTION('center_axis',(0.,-1.,0.));
#10912=DIRECTION('ref_axis',(0.,0.,-1.));
#10913=DIRECTION('center_axis',(0.,0.,1.));
#10914=DIRECTION('ref_axis',(1.,0.,0.));
#10915=DIRECTION('center_axis',(0.,-1.,0.));
#10916=DIRECTION('ref_axis',(0.,0.,-1.));
#10917=DIRECTION('center_axis',(0.,-1.,0.));
#10918=DIRECTION('ref_axis',(-1.,0.,0.));
#10919=DIRECTION('center_axis',(0.,1.,0.));
#10920=DIRECTION('ref_axis',(1.,0.,0.));
#13504=CARTESIAN_POINT('',(0.,0.,0.));
#13505=CARTESIAN_POINT('Origin',(1.47463555300403,0.,1.23736614864659));
#13506=CARTESIAN_POINT('',(1.16188454446795,-0.07938,1.49479506783723));
#13507=CARTESIAN_POINT('',(1.67384490577674,-0.07938,0.884664467981643));
#13508=CARTESIAN_POINT('Ctrl Pts',(1.16188454446795,-0.07938,1.49479506783723));
#13509=CARTESIAN_POINT('Ctrl Pts',(1.16869700612251,-0.123392992551698,
1.48949983100074));
#13510=CARTESIAN_POINT('Ctrl Pts',(1.18135446441955,-0.166529565724166,
1.47962830891229));
#13511=CARTESIAN_POINT('Ctrl Pts',(1.21282145231718,-0.237213819614884,
1.45388393800011));
#13512=CARTESIAN_POINT('Ctrl Pts',(1.22989120215288,-0.266247928944116,
1.4395843844684));
#13513=CARTESIAN_POINT('Ctrl Pts',(1.26813946847809,-0.317173992396757,
1.40600777299249));
#13514=CARTESIAN_POINT('Ctrl Pts',(1.28931069477441,-0.339063173951852,
1.38671820696899));
#13515=CARTESIAN_POINT('Ctrl Pts',(1.33224261954459,-0.373566122196588,
1.34549913552853));
#13516=CARTESIAN_POINT('Ctrl Pts',(1.35618281536764,-0.388075792674378,
1.32151296077672));
#13517=CARTESIAN_POINT('Ctrl Pts',(1.40439359896051,-0.407069005705619,
1.27016020894803));
#13518=CARTESIAN_POINT('Ctrl Pts',(1.42864614483643,-0.411552957311693,
1.24277684810113));
#13519=CARTESIAN_POINT('Ctrl Pts',(1.4719780748558,-0.411552957311693,1.19113586482651));
#13520=CARTESIAN_POINT('Ctrl Pts',(1.49473401052622,-0.407069005705619,
1.16249669890816));
#13521=CARTESIAN_POINT('Ctrl Pts',(1.53693488395083,-0.388075792674377,
1.10610103367387));
#13522=CARTESIAN_POINT('Ctrl Pts',(1.55639948343386,-0.373566122196588,
1.07835938768384));
#13523=CARTESIAN_POINT('Ctrl Pts',(1.58953729406031,-0.339063173951852,
1.02892207867768));
#13524=CARTESIAN_POINT('Ctrl Pts',(1.60485746336717,-0.317173992396757,
1.00472289289232));
#13525=CARTESIAN_POINT('Ctrl Pts',(1.63128222892223,-0.266247928944116,
0.961225186280959));
#13526=CARTESIAN_POINT('Ctrl Pts',(1.64240040915267,-0.237213819614884,
0.941931672888549));
#13527=CARTESIAN_POINT('Ctrl Pts',(1.66228948011831,-0.166529565724165,
0.906472276148935));
#13528=CARTESIAN_POINT('Ctrl Pts',(1.66981308703787,-0.123392992551698,
0.892292941263125));
#13529=CARTESIAN_POINT('Ctrl Pts',(1.67384490577674,-0.07938,0.884664467981643));
#13530=CARTESIAN_POINT('',(1.20622598189858,-0.07938,1.54074568637942));
#13531=CARTESIAN_POINT('Origin',(1.47463555300403,-0.07938,1.23736614864659));
#13532=CARTESIAN_POINT('',(1.72679724097776,-0.07938,0.920353018170519));
#13533=CARTESIAN_POINT('Ctrl Pts',(1.72679724097776,-0.0793800000000002,
0.920353018170518));
#13534=CARTESIAN_POINT('Ctrl Pts',(1.72470909046691,-0.10165971810728,0.92427087628551));
#13535=CARTESIAN_POINT('Ctrl Pts',(1.72169532435455,-0.123845306465941,
0.929898398578877));
#13536=CARTESIAN_POINT('Ctrl Pts',(1.70911544962889,-0.192537547974292,
0.952957916220029));
#13537=CARTESIAN_POINT('Ctrl Pts',(1.69580594901181,-0.236239311587943,
0.976785804874841));
#13538=CARTESIAN_POINT('Ctrl Pts',(1.66527150643903,-0.303218781300911,
1.02787962443771));
#13539=CARTESIAN_POINT('Ctrl Pts',(1.64438322958071,-0.3351607303803,1.06123747122987));
#13540=CARTESIAN_POINT('Ctrl Pts',(1.60730731395783,-0.3732673312795,1.11639170354769));
#13541=CARTESIAN_POINT('Ctrl Pts',(1.5873911192195,-0.387903357081022,1.1447096804553));
#13542=CARTESIAN_POINT('Ctrl Pts',(1.54427174765086,-0.40704475551587,1.20224605970712));
#13543=CARTESIAN_POINT('Ctrl Pts',(1.52104964294098,-0.411552957311693,
1.23144933316771));
#13544=CARTESIAN_POINT('Ctrl Pts',(1.47686834938291,-0.411552957311693,
1.284102548491));
#13545=CARTESIAN_POINT('Ctrl Pts',(1.45214121543005,-0.40704475551587,1.31204295246889));
#13546=CARTESIAN_POINT('Ctrl Pts',(1.40296654335764,-0.387903357081022,
1.36449833130133));
#13547=CARTESIAN_POINT('Ctrl Pts',(1.37853719107178,-0.3732673312795,1.38902931937536));
#13548=CARTESIAN_POINT('Ctrl Pts',(1.330659040657,-0.3351607303803,1.43511940046341));
#13549=CARTESIAN_POINT('Ctrl Pts',(1.30143518572334,-0.303218781300911,
1.4614828667669));
#13550=CARTESIAN_POINT('Ctrl Pts',(1.25641984639565,-0.236239311587943,
1.50042577120361));
#13551=CARTESIAN_POINT('Ctrl Pts',(1.23526512743829,-0.192537547974292,
1.51767074004259));
#13552=CARTESIAN_POINT('Ctrl Pts',(1.21474040800595,-0.123845306465941,
1.53406374142061));
#13553=CARTESIAN_POINT('Ctrl Pts',(1.20972171541452,-0.10165971810728,1.53800893064485));
#13554=CARTESIAN_POINT('Ctrl Pts',(1.20622598189858,-0.0793800000000002,
1.54074568637942));
#13555=CARTESIAN_POINT('Origin',(1.47463555300403,-0.07938,1.23736614864659));
#13556=CARTESIAN_POINT('Origin',(0.,-0.27783,0.));
#13557=CARTESIAN_POINT('',(0.731211914226578,-0.07938,1.81499518621871));
#13558=CARTESIAN_POINT('Origin',(0.,-0.07938,0.));
#13559=CARTESIAN_POINT('',(-0.0663495263035324,-0.07938,1.95562678695688));
#13560=CARTESIAN_POINT('Ctrl Pts',(0.73121191422658,-0.0793800000000002,
1.81499518621871));
#13561=CARTESIAN_POINT('Ctrl Pts',(0.727093947478514,-0.10165971810728,
1.81665420238109));
#13562=CARTESIAN_POINT('Ctrl Pts',(0.721167967091869,-0.123845306465941,
1.81902792304693));
#13563=CARTESIAN_POINT('Ctrl Pts',(0.696708851738065,-0.192537547974292,
1.82860635079188));
#13564=CARTESIAN_POINT('Ctrl Pts',(0.671196911157359,-0.236239311587943,
1.83830439039938));
#13565=CARTESIAN_POINT('Ctrl Pts',(0.614963696954177,-0.303218781300911,
1.85781736559878));
#13566=CARTESIAN_POINT('Ctrl Pts',(0.577520337936704,-0.3351607303803,1.86994423321609));
#13567=CARTESIAN_POINT('Ctrl Pts',(0.513666081644577,-0.3732673312795,1.88836288721748));
#13568=CARTESIAN_POINT('Ctrl Pts',(0.48020694664961,-0.387903357081022,
1.89725383285802));
#13569=CARTESIAN_POINT('Ctrl Pts',(0.410191919979371,-0.40704475551587,
1.91361265867928));
#13570=CARTESIAN_POINT('Ctrl Pts',(0.373631253366087,-0.411552957311693,
1.92105678285629));
#13571=CARTESIAN_POINT('Ctrl Pts',(0.305941584526154,-0.411552957311693,
1.932992297788));
#13572=CARTESIAN_POINT('Ctrl Pts',(0.269039755480681,-0.40704475551587,
1.9385015936658));
#13573=CARTESIAN_POINT('Ctrl Pts',(0.197652103622503,-0.387903357081022,
1.94707587521355));
#13574=CARTESIAN_POINT('Ctrl Pts',(0.163169918867575,-0.3732673312795,1.95016481734985));
#13575=CARTESIAN_POINT('Ctrl Pts',(0.09686699474267,-0.3351607303803,1.95469638598893));
#13576=CARTESIAN_POINT('Ctrl Pts',(0.0575341135759475,-0.30321878130091,
1.95610724099344));
#13577=CARTESIAN_POINT('Ctrl Pts',(-0.00198165342826295,-0.236239311587942,
1.95700393417042));
#13578=CARTESIAN_POINT('Ctrl Pts',(-0.0292719606304177,-0.192537547974292,
1.95661635548909));
#13579=CARTESIAN_POINT('Ctrl Pts',(-0.0555320260694991,-0.123845306465941,
1.95598108775736));
#13580=CARTESIAN_POINT('Ctrl Pts',(-0.0619124863920986,-0.10165971810728,
1.95577732462505));
#13581=CARTESIAN_POINT('Ctrl Pts',(-0.0663495263035336,-0.0793800000000002,
1.95562678695688));
#13582=CARTESIAN_POINT('',(-0.606515593706441,-0.07938,1.86038093521056));
#13583=CARTESIAN_POINT('Origin',(0.,-0.07938,0.));
#13584=CARTESIAN_POINT('',(-1.30787935375538,-0.07938,1.45544837954646));
#13585=CARTESIAN_POINT('Ctrl Pts',(-0.60651559370644,-0.0793800000000002,
1.86038093521056));
#13586=CARTESIAN_POINT('Ctrl Pts',(-0.610736534284191,-0.10165971810728,
1.85900483732004));
#13587=CARTESIAN_POINT('Ctrl Pts',(-0.616801896862274,-0.123845306465941,
1.85701406607784));
#13588=CARTESIAN_POINT('Ctrl Pts',(-0.64169556093739,-0.192537547974292,
1.84862955113236));
#13589=CARTESIAN_POINT('Ctrl Pts',(-0.667472620950374,-0.236239311587943,
1.8396599211785));
#13590=CARTESIAN_POINT('Ctrl Pts',(-0.723092460895733,-0.303218781300911,
1.81846171405606));
#13591=CARTESIAN_POINT('Ctrl Pts',(-0.759570738251496,-0.3351607303803,
1.80368330636526));
#13592=CARTESIAN_POINT('Ctrl Pts',(-0.820325219032771,-0.3732673312795,
1.77674808914243));
#13593=CARTESIAN_POINT('Ctrl Pts',(-0.851671393163369,-0.387903357081022,
1.76205183123884));
#13594=CARTESIAN_POINT('Ctrl Pts',(-0.915821265825857,-0.40704475551587,
1.72957862721967));
#13595=CARTESIAN_POINT('Ctrl Pts',(-0.948613352107641,-0.411552957311693,
1.71178041367846));
#13596=CARTESIAN_POINT('Ctrl Pts',(-1.00813864789236,-0.411552957311693,
1.67741346813356));
#13597=CARTESIAN_POINT('Ctrl Pts',(-1.03994839610192,-0.40704475551587,
1.65791379514105));
#13598=CARTESIAN_POINT('Ctrl Pts',(-1.10014595205605,-0.387903357081022,
1.61859497777538));
#13599=CARTESIAN_POINT('Ctrl Pts',(-1.12854637180642,-0.3732673312795,1.59879652361863));
#13600=CARTESIAN_POINT('Ctrl Pts',(-1.18225019456848,-0.3351607303803,1.55964920847973));
#13601=CARTESIAN_POINT('Ctrl Pts',(-1.21328780973407,-0.30321878130091,
1.53544729744874));
#13602=CARTESIAN_POINT('Ctrl Pts',(-1.25945591558947,-0.236239311587942,
1.49787820666285));
#13603=CARTESIAN_POINT('Ctrl Pts',(-1.28011237299855,-0.192537547974292,
1.48003943283366));
#13604=CARTESIAN_POINT('Ctrl Pts',(-1.29982040797731,-0.12384530646594,
1.46267314482408));
#13605=CARTESIAN_POINT('Ctrl Pts',(-1.30457714773522,-0.10165971810728,
1.45841577236939));
#13606=CARTESIAN_POINT('Ctrl Pts',(-1.30787935375538,-0.0793800000000002,
1.45544837954646));
#13607=CARTESIAN_POINT('',(-1.66044771467423,-0.07938,1.03527376878636));
#13608=CARTESIAN_POINT('Origin',(0.,-0.07938,0.));
#13609=CARTESIAN_POINT('',(-1.93743789612516,-0.07938,0.274249499839291));
#13610=CARTESIAN_POINT('Ctrl Pts',(-1.66044771467423,-0.0793800000000002,
1.03527376878636));
#13611=CARTESIAN_POINT('Ctrl Pts',(-1.66279660407481,-0.10165971810728,
1.03150644833954));
#13612=CARTESIAN_POINT('Ctrl Pts',(-1.66616329828505,-0.123845306465941,
1.02608268917849));
#13613=CARTESIAN_POINT('Ctrl Pts',(-1.67984348899847,-0.192537547974292,
1.00365843926907));
#13614=CARTESIAN_POINT('Ctrl Pts',(-1.69382429558355,-0.236239311587943,
0.980218129295584));
#13615=CARTESIAN_POINT('Ctrl Pts',(-1.72280562001498,-0.303218781300911,
0.928227616555729));
#13616=CARTESIAN_POINT('Ctrl Pts',(-1.74125022432338,-0.3351607303803,0.893458914759057));
#13617=CARTESIAN_POINT('Ctrl Pts',(-1.7704772328254,-0.3732673312795,0.833773113802161));
#13618=CARTESIAN_POINT('Ctrl Pts',(-1.785043222842,-0.387903357081022,0.802366194758251));
#13619=CARTESIAN_POINT('Ctrl Pts',(-1.81331150313154,-0.407044755515871,
0.736255533958675));
#13620=CARTESIAN_POINT('Ctrl Pts',(-1.82699122746714,-0.411552957311693,
0.701542964620283));
#13621=CARTESIAN_POINT('Ctrl Pts',(-1.850499602749,-0.411552957311693,0.636954234365294));
#13622=CARTESIAN_POINT('Ctrl Pts',(-1.86233313540942,-0.40704475551587,
0.60156970621039));
#13623=CARTESIAN_POINT('Ctrl Pts',(-1.88317349000725,-0.387903357081022,
0.53275550155669));
#13624=CARTESIAN_POINT('Ctrl Pts',(-1.89220327271636,-0.3732673312795,0.499333567842125));
#13625=CARTESIAN_POINT('Ctrl Pts',(-1.9081793785937,-0.3351607303803,0.434824832752687));
#13626=CARTESIAN_POINT('Ctrl Pts',(-1.91639888267751,-0.30321878130091,
0.396334498831876));
#13627=CARTESIAN_POINT('Ctrl Pts',(-1.92761675755301,-0.236239311587942,
0.337878619195771));
#13628=CARTESIAN_POINT('Ctrl Pts',(-1.93197397917636,-0.192537547974292,
0.310935610749289));
#13629=CARTESIAN_POINT('Ctrl Pts',(-1.93590837509782,-0.12384530646594,
0.284964181626328));
#13630=CARTESIAN_POINT('Ctrl Pts',(-1.93681566289304,-0.10165971810728,
0.278645271736243));
#13631=CARTESIAN_POINT('Ctrl Pts',(-1.93743789612516,-0.0793800000000002,
0.27424949983929));
#13632=CARTESIAN_POINT('',(-1.956752,-0.07938,2.39633007352518E-16));
#13633=CARTESIAN_POINT('Origin',(0.,-0.07938,0.));
#13634=CARTESIAN_POINT('',(-1.956752,-0.47628,2.39633007352518E-16));
#13635=CARTESIAN_POINT('',(-1.956752,-0.27783,2.39633007352518E-16));
#13636=CARTESIAN_POINT('Origin',(0.,-0.47628,0.));
#13637=CARTESIAN_POINT('',(-1.93743789612516,-0.07938,-0.274249499839292));
#13638=CARTESIAN_POINT('Origin',(0.,-0.07938,0.));
#13639=CARTESIAN_POINT('',(-1.66044771467423,-0.07938,-1.03527376878636));
#13640=CARTESIAN_POINT('Ctrl Pts',(-1.93743789612516,-0.0793800000000002,
-0.27424949983929));
#13641=CARTESIAN_POINT('Ctrl Pts',(-1.93681566289304,-0.10165971810728,
-0.278645271736244));
#13642=CARTESIAN_POINT('Ctrl Pts',(-1.93590837509782,-0.123845306465941,
-0.284964181626328));
#13643=CARTESIAN_POINT('Ctrl Pts',(-1.93197397917636,-0.192537547974292,
-0.310935610749289));
#13644=CARTESIAN_POINT('Ctrl Pts',(-1.92761675755301,-0.236239311587942,
-0.337878619195772));
#13645=CARTESIAN_POINT('Ctrl Pts',(-1.91639888267751,-0.303218781300911,
-0.396334498831877));
#13646=CARTESIAN_POINT('Ctrl Pts',(-1.9081793785937,-0.3351607303803,-0.434824832752687));
#13647=CARTESIAN_POINT('Ctrl Pts',(-1.89220327271636,-0.3732673312795,-0.499333567842125));
#13648=CARTESIAN_POINT('Ctrl Pts',(-1.88317349000725,-0.387903357081022,
-0.53275550155669));
#13649=CARTESIAN_POINT('Ctrl Pts',(-1.86233313540942,-0.40704475551587,
-0.601569706210391));
#13650=CARTESIAN_POINT('Ctrl Pts',(-1.850499602749,-0.411552957311693,-0.636954234365295));
#13651=CARTESIAN_POINT('Ctrl Pts',(-1.82699122746714,-0.411552957311693,
-0.701542964620284));
#13652=CARTESIAN_POINT('Ctrl Pts',(-1.81331150313154,-0.40704475551587,
-0.736255533958675));
#13653=CARTESIAN_POINT('Ctrl Pts',(-1.785043222842,-0.387903357081022,-0.802366194758251));
#13654=CARTESIAN_POINT('Ctrl Pts',(-1.7704772328254,-0.3732673312795,-0.833773113802161));
#13655=CARTESIAN_POINT('Ctrl Pts',(-1.74125022432338,-0.3351607303803,-0.893458914759057));
#13656=CARTESIAN_POINT('Ctrl Pts',(-1.72280562001498,-0.303218781300911,
-0.92822761655573));
#13657=CARTESIAN_POINT('Ctrl Pts',(-1.69382429558355,-0.236239311587942,
-0.980218129295584));
#13658=CARTESIAN_POINT('Ctrl Pts',(-1.67984348899847,-0.192537547974292,
-1.00365843926907));
#13659=CARTESIAN_POINT('Ctrl Pts',(-1.66616329828505,-0.123845306465941,
-1.02608268917849));
#13660=CARTESIAN_POINT('Ctrl Pts',(-1.66279660407481,-0.10165971810728,
-1.03150644833954));
#13661=CARTESIAN_POINT('Ctrl Pts',(-1.66044771467423,-0.0793800000000001,
-1.03527376878636));
#13662=CARTESIAN_POINT('',(-1.30787935375538,-0.07938,-1.45544837954646));
#13663=CARTESIAN_POINT('Origin',(0.,-0.07938,0.));
#13664=CARTESIAN_POINT('',(-0.60651559370644,-0.07938,-1.86038093521056));
#13665=CARTESIAN_POINT('Ctrl Pts',(-1.30787935375538,-0.0793800000000002,
-1.45544837954646));
#13666=CARTESIAN_POINT('Ctrl Pts',(-1.30457714773522,-0.10165971810728,
-1.45841577236939));
#13667=CARTESIAN_POINT('Ctrl Pts',(-1.29982040797731,-0.123845306465941,
-1.46267314482408));
#13668=CARTESIAN_POINT('Ctrl Pts',(-1.28011237299855,-0.192537547974292,
-1.48003943283366));
#13669=CARTESIAN_POINT('Ctrl Pts',(-1.25945591558947,-0.236239311587942,
-1.49787820666285));
#13670=CARTESIAN_POINT('Ctrl Pts',(-1.21328780973407,-0.303218781300911,
-1.53544729744874));
#13671=CARTESIAN_POINT('Ctrl Pts',(-1.18225019456848,-0.3351607303803,-1.55964920847973));
#13672=CARTESIAN_POINT('Ctrl Pts',(-1.12854637180642,-0.3732673312795,-1.59879652361863));
#13673=CARTESIAN_POINT('Ctrl Pts',(-1.10014595205605,-0.387903357081022,
-1.61859497777538));
#13674=CARTESIAN_POINT('Ctrl Pts',(-1.03994839610192,-0.40704475551587,
-1.65791379514105));
#13675=CARTESIAN_POINT('Ctrl Pts',(-1.00813864789236,-0.411552957311693,
-1.67741346813356));
#13676=CARTESIAN_POINT('Ctrl Pts',(-0.948613352107639,-0.411552957311693,
-1.71178041367846));
#13677=CARTESIAN_POINT('Ctrl Pts',(-0.915821265825855,-0.40704475551587,
-1.72957862721967));
#13678=CARTESIAN_POINT('Ctrl Pts',(-0.851671393163367,-0.387903357081022,
-1.76205183123885));
#13679=CARTESIAN_POINT('Ctrl Pts',(-0.820325219032769,-0.3732673312795,
-1.77674808914243));
#13680=CARTESIAN_POINT('Ctrl Pts',(-0.759570738251494,-0.3351607303803,
-1.80368330636526));
#13681=CARTESIAN_POINT('Ctrl Pts',(-0.723092460895731,-0.303218781300911,
-1.81846171405606));
#13682=CARTESIAN_POINT('Ctrl Pts',(-0.667472620950373,-0.236239311587942,
-1.8396599211785));
#13683=CARTESIAN_POINT('Ctrl Pts',(-0.641695560937389,-0.192537547974292,
-1.84862955113236));
#13684=CARTESIAN_POINT('Ctrl Pts',(-0.616801896862272,-0.123845306465941,
-1.85701406607784));
#13685=CARTESIAN_POINT('Ctrl Pts',(-0.610736534284189,-0.10165971810728,
-1.85900483732004));
#13686=CARTESIAN_POINT('Ctrl Pts',(-0.606515593706439,-0.0793800000000002,
-1.86038093521056));
#13687=CARTESIAN_POINT('',(-0.0663495263035315,-0.07938,-1.95562678695688));
#13688=CARTESIAN_POINT('Origin',(0.,-0.07938,0.));
#13689=CARTESIAN_POINT('',(0.731211914226579,-0.07938,-1.81499518621871));
#13690=CARTESIAN_POINT('Ctrl Pts',(-0.0663495263035327,-0.0793800000000002,
-1.95562678695688));
#13691=CARTESIAN_POINT('Ctrl Pts',(-0.0619124863920977,-0.10165971810728,
-1.95577732462505));
#13692=CARTESIAN_POINT('Ctrl Pts',(-0.0555320260694982,-0.123845306465941,
-1.95598108775736));
#13693=CARTESIAN_POINT('Ctrl Pts',(-0.0292719606304167,-0.192537547974292,
-1.95661635548909));
#13694=CARTESIAN_POINT('Ctrl Pts',(-0.00198165342826177,-0.236239311587943,
-1.95700393417042));
#13695=CARTESIAN_POINT('Ctrl Pts',(0.0575341135759488,-0.303218781300911,
-1.95610724099344));
#13696=CARTESIAN_POINT('Ctrl Pts',(0.0968669947426714,-0.3351607303803,
-1.95469638598893));
#13697=CARTESIAN_POINT('Ctrl Pts',(0.163169918867576,-0.3732673312795,-1.95016481734985));
#13698=CARTESIAN_POINT('Ctrl Pts',(0.197652103622504,-0.387903357081022,
-1.94707587521355));
#13699=CARTESIAN_POINT('Ctrl Pts',(0.269039755480682,-0.40704475551587,
-1.9385015936658));
#13700=CARTESIAN_POINT('Ctrl Pts',(0.305941584526155,-0.411552957311693,
-1.93299229778799));
#13701=CARTESIAN_POINT('Ctrl Pts',(0.373631253366089,-0.411552957311693,
-1.92105678285629));
#13702=CARTESIAN_POINT('Ctrl Pts',(0.410191919979372,-0.40704475551587,
-1.91361265867928));
#13703=CARTESIAN_POINT('Ctrl Pts',(0.480206946649611,-0.387903357081022,
-1.89725383285802));
#13704=CARTESIAN_POINT('Ctrl Pts',(0.513666081644578,-0.3732673312795,-1.88836288721748));
#13705=CARTESIAN_POINT('Ctrl Pts',(0.577520337936705,-0.3351607303803,-1.86994423321609));
#13706=CARTESIAN_POINT('Ctrl Pts',(0.614963696954178,-0.30321878130091,
-1.85781736559878));
#13707=CARTESIAN_POINT('Ctrl Pts',(0.67119691115736,-0.236239311587942,
-1.83830439039938));
#13708=CARTESIAN_POINT('Ctrl Pts',(0.696708851738067,-0.192537547974292,
-1.82860635079188));
#13709=CARTESIAN_POINT('Ctrl Pts',(0.721167967091869,-0.123845306465941,
-1.81902792304693));
#13710=CARTESIAN_POINT('Ctrl Pts',(0.727093947478515,-0.10165971810728,
-1.81665420238109));
#13711=CARTESIAN_POINT('Ctrl Pts',(0.73121191422658,-0.0793800000000002,
-1.81499518621871));
#13712=CARTESIAN_POINT('',(1.20622598189858,-0.07938,-1.54074568637942));
#13713=CARTESIAN_POINT('Origin',(0.,-0.07938,0.));
#13714=CARTESIAN_POINT('',(1.72679724097776,-0.07938,-0.920353018170518));
#13715=CARTESIAN_POINT('Ctrl Pts',(1.20622598189858,-0.0793800000000002,
-1.54074568637942));
#13716=CARTESIAN_POINT('Ctrl Pts',(1.20972171541452,-0.10165971810728,-1.53800893064485));
#13717=CARTESIAN_POINT('Ctrl Pts',(1.21474040800596,-0.123845306465941,
-1.53406374142061));
#13718=CARTESIAN_POINT('Ctrl Pts',(1.23526512743829,-0.192537547974292,
-1.51767074004259));
#13719=CARTESIAN_POINT('Ctrl Pts',(1.25641984639565,-0.236239311587942,
-1.50042577120361));
#13720=CARTESIAN_POINT('Ctrl Pts',(1.30143518572334,-0.303218781300911,
-1.4614828667669));
#13721=CARTESIAN_POINT('Ctrl Pts',(1.330659040657,-0.3351607303803,-1.43511940046341));
#13722=CARTESIAN_POINT('Ctrl Pts',(1.37853719107178,-0.3732673312795,-1.38902931937536));
#13723=CARTESIAN_POINT('Ctrl Pts',(1.40296654335764,-0.387903357081022,
-1.36449833130133));
#13724=CARTESIAN_POINT('Ctrl Pts',(1.45214121543005,-0.40704475551587,-1.31204295246889));
#13725=CARTESIAN_POINT('Ctrl Pts',(1.47686834938291,-0.411552957311693,
-1.284102548491));
#13726=CARTESIAN_POINT('Ctrl Pts',(1.52104964294098,-0.411552957311693,
-1.23144933316771));
#13727=CARTESIAN_POINT('Ctrl Pts',(1.54427174765086,-0.407044755515871,
-1.20224605970712));
#13728=CARTESIAN_POINT('Ctrl Pts',(1.5873911192195,-0.387903357081022,-1.1447096804553));
#13729=CARTESIAN_POINT('Ctrl Pts',(1.60730731395783,-0.3732673312795,-1.11639170354769));
#13730=CARTESIAN_POINT('Ctrl Pts',(1.64438322958071,-0.3351607303803,-1.06123747122987));
#13731=CARTESIAN_POINT('Ctrl Pts',(1.66527150643903,-0.303218781300911,
-1.02787962443771));
#13732=CARTESIAN_POINT('Ctrl Pts',(1.69580594901181,-0.236239311587943,
-0.976785804874841));
#13733=CARTESIAN_POINT('Ctrl Pts',(1.70911544962889,-0.192537547974292,
-0.952957916220028));
#13734=CARTESIAN_POINT('Ctrl Pts',(1.72169532435455,-0.123845306465941,
-0.929898398578876));
#13735=CARTESIAN_POINT('Ctrl Pts',(1.72470909046691,-0.10165971810728,-0.924270876285509));
#13736=CARTESIAN_POINT('Ctrl Pts',(1.72679724097776,-0.0793800000000002,
-0.920353018170518));
#13737=CARTESIAN_POINT('',(1.91439494746182,-0.07938,-0.404932555664102));
#13738=CARTESIAN_POINT('Origin',(0.,-0.07938,0.));
#13739=CARTESIAN_POINT('',(1.91439494746182,-0.07938,0.404932555664102));
#13740=CARTESIAN_POINT('Ctrl Pts',(1.91439494746182,-0.0793800000000002,
-0.404932555664103));
#13741=CARTESIAN_POINT('Ctrl Pts',(1.91531368201941,-0.10165971810728,-0.400589064950645));
#13742=CARTESIAN_POINT('Ctrl Pts',(1.91662230483958,-0.123845306465941,
-0.394340921253764));
#13743=CARTESIAN_POINT('Ctrl Pts',(1.92180793393594,-0.192537547974292,
-0.368590118298695));
#13744=CARTESIAN_POINT('Ctrl Pts',(1.92692853653984,-0.236239311587943,
-0.341781714515643));
#13745=CARTESIAN_POINT('Ctrl Pts',(1.9363802706298,-0.303218781300911,-0.283014416607319));
#13746=CARTESIAN_POINT('Ctrl Pts',(1.94182093281998,-0.3351607303803,-0.244034097885537));
#13747=CARTESIAN_POINT('Ctrl Pts',(1.94887159083919,-0.3732673312795,-0.177951565523803));
#13748=CARTESIAN_POINT('Ctrl Pts',(1.95181734521941,-0.387903357081022,
-0.143456853463462));
#13749=CARTESIAN_POINT('Ctrl Pts',(1.95576966192778,-0.40704475551587,-0.071664832078622));
#13750=CARTESIAN_POINT('Ctrl Pts',(1.956752,-0.411552957311693,-0.0343669455449008));
#13751=CARTESIAN_POINT('Ctrl Pts',(1.956752,-0.411552957311693,0.0343669455449008));
#13752=CARTESIAN_POINT('Ctrl Pts',(1.95576966192778,-0.40704475551587,0.0716648320786219));
#13753=CARTESIAN_POINT('Ctrl Pts',(1.95181734521941,-0.387903357081022,
0.143456853463462));
#13754=CARTESIAN_POINT('Ctrl Pts',(1.94887159083919,-0.3732673312795,0.177951565523803));
#13755=CARTESIAN_POINT('Ctrl Pts',(1.94182093281998,-0.3351607303803,0.244034097885537));
#13756=CARTESIAN_POINT('Ctrl Pts',(1.9363802706298,-0.303218781300911,0.283014416607319));
#13757=CARTESIAN_POINT('Ctrl Pts',(1.92692853653984,-0.236239311587943,
0.341781714515643));
#13758=CARTESIAN_POINT('Ctrl Pts',(1.92180793393594,-0.192537547974292,
0.368590118298695));
#13759=CARTESIAN_POINT('Ctrl Pts',(1.91662230483958,-0.123845306465941,
0.394340921253764));
#13760=CARTESIAN_POINT('Ctrl Pts',(1.91531368201941,-0.10165971810728,0.400589064950645));
#13761=CARTESIAN_POINT('Ctrl Pts',(1.91439494746182,-0.0793800000000002,
0.404932555664103));
#13762=CARTESIAN_POINT('Origin',(0.,-0.07938,0.));
#13763=CARTESIAN_POINT('Origin',(0.,-0.07938,0.));
#13764=CARTESIAN_POINT('',(0.71358822996475,-0.07938,1.75361906569237));
#13765=CARTESIAN_POINT('Origin',(0.,-0.07938,0.));
#13766=CARTESIAN_POINT('Origin',(0.33427274200884,-0.07938,1.8957549245485));
#13767=CARTESIAN_POINT('Origin',(0.33427274200884,0.,1.8957549245485));
#13768=CARTESIAN_POINT('',(-0.070780549790825,-0.07938,1.89192444438865));
#13769=CARTESIAN_POINT('Ctrl Pts',(-0.0707805497908251,-0.07938,1.89192444438865));
#13770=CARTESIAN_POINT('Ctrl Pts',(-0.0621581887675352,-0.123392992551698,
1.89224702357808));
#13771=CARTESIAN_POINT('Ctrl Pts',(-0.0461167210878756,-0.166529565724166,
1.89282105630055));
#13772=CARTESIAN_POINT('Ctrl Pts',(-0.00546344722567869,-0.237213819614884,
1.89332631395644));
#13773=CARTESIAN_POINT('Ctrl Pts',(0.0168043156156246,-0.266247928944116,
1.89334444412923));
#13774=CARTESIAN_POINT('Ctrl Pts',(0.0676868173249578,-0.317173992396757,
1.89220877917518));
#13775=CARTESIAN_POINT('Ctrl Pts',(0.0963040116194015,-0.339063173951852,
1.89104071625784));
#13776=CARTESIAN_POINT('Ctrl Pts',(0.155686882426711,-0.373566122196588,
1.88706118493262));
#13777=CARTESIAN_POINT('Ctrl Pts',(0.189444152338378,-0.388075792674378,
1.88407517030084));
#13778=CARTESIAN_POINT('Ctrl Pts',(0.259384667806906,-0.407069005705619,
1.87572597447038));
#13779=CARTESIAN_POINT('Ctrl Pts',(0.295564880870602,-0.411552957311693,
1.87033833905209));
#13780=CARTESIAN_POINT('Ctrl Pts',(0.361953249272518,-0.411552957311693,
1.85863227849762));
#13781=CARTESIAN_POINT('Ctrl Pts',(0.397794208344885,-0.407069005705619,
1.85132063808607));
#13782=CARTESIAN_POINT('Ctrl Pts',(0.466372387779211,-0.388075792674377,
1.83524525067264));
#13783=CARTESIAN_POINT('Ctrl Pts',(0.499115122365417,-0.373566122196588,
1.82650552029421));
#13784=CARTESIAN_POINT('Ctrl Pts',(0.55627784773835,-0.339063173951852,
1.8099349185301));
#13785=CARTESIAN_POINT('Ctrl Pts',(0.583568715090836,-0.317173992396757,
1.80124488173997));
#13786=CARTESIAN_POINT('Ctrl Pts',(0.631771046764577,-0.266247928944116,
1.78490921718958));
#13787=CARTESIAN_POINT('Ctrl Pts',(0.652689698303665,-0.237213819614884,
1.77727615696148));
#13788=CARTESIAN_POINT('Ctrl Pts',(0.690718471466875,-0.166529565724165,
1.76289713151763));
#13789=CARTESIAN_POINT('Ctrl Pts',(0.705596189518013,-0.123392992551698,
1.75687121212928));
#13790=CARTESIAN_POINT('Ctrl Pts',(0.71358822996475,-0.07938,1.75361906569237));
#13791=CARTESIAN_POINT('Origin',(0.33427274200884,-0.07938,1.8957549245485));
#13792=CARTESIAN_POINT('Origin',(0.,-0.07938,0.));
#13793=CARTESIAN_POINT('',(-0.580564309297537,-0.07938,1.80203581326062));
#13794=CARTESIAN_POINT('Origin',(0.,-0.07938,0.));
#13795=CARTESIAN_POINT('Origin',(-0.962500000000001,-0.07938,1.66709890228504));
#13796=CARTESIAN_POINT('Origin',(-0.962500000000001,0.,1.66709890228504));
#13797=CARTESIAN_POINT('',(-1.27032663816428,-0.07938,1.40380134701254));
#13798=CARTESIAN_POINT('Ctrl Pts',(-1.27032663816428,-0.07938,1.40380134701254));
#13799=CARTESIAN_POINT('Ctrl Pts',(-1.26392887632193,-0.123392992551698,
1.40959080384008));
#13800=CARTESIAN_POINT('Ctrl Pts',(-1.25200938026802,-0.166529565724166,
1.42034179508297));
#13801=CARTESIAN_POINT('Ctrl Pts',(-1.22119193909219,-0.237213819614885,
1.44686026563443));
#13802=CARTESIAN_POINT('Ctrl Pts',(-1.20414549695735,-0.266247928944117,
1.46118759620237));
#13803=CARTESIAN_POINT('Ctrl Pts',(-1.16443724790971,-0.317173992396758,
1.49302426802369));
#13804=CARTESIAN_POINT('Ctrl Pts',(-1.14176438887219,-0.339063173951853,
1.51052425783311));
#13805=CARTESIAN_POINT('Ctrl Pts',(-1.09371647724559,-0.373566122196589,
1.54564633355776));
#13806=CARTESIAN_POINT('Ctrl Pts',(-1.06593753500724,-0.388075792674378,
1.56505766847808));
#13807=CARTESIAN_POINT('Ctrl Pts',(-1.00699323215303,-0.407069005705619,
1.6036187101659));
#13808=CARTESIAN_POINT('Ctrl Pts',(-0.975814475692339,-0.411552957311693,
1.62274773466534));
#13809=CARTESIAN_POINT('Ctrl Pts',(-0.917433524307661,-0.411552957311693,
1.65645399266283));
#13810=CARTESIAN_POINT('Ctrl Pts',(-0.885277924911194,-0.407069005705619,
1.67389107556648));
#13811=CARTESIAN_POINT('Ctrl Pts',(-0.822410931786043,-0.388075792674377,
1.70565781840267));
#13812=CARTESIAN_POINT('Ctrl Pts',(-0.791710751504505,-0.373566122196588,
1.72000942061118));
#13813=CARTESIAN_POINT('Ctrl Pts',(-0.737270185880016,-0.339063173951852,
1.74405909481629));
#13814=CARTESIAN_POINT('Ctrl Pts',(-0.710778320620332,-0.317173992396757,
1.75494437181449));
#13815=CARTESIAN_POINT('Ctrl Pts',(-0.663352829527299,-0.266247928944116,
1.77341438831889));
#13816=CARTESIAN_POINT('Ctrl Pts',(-0.642421776219621,-0.237213819614884,
1.78101337496783));
#13817=CARTESIAN_POINT('Ctrl Pts',(-0.604047386464641,-0.166529565724165,
1.79444282663));
#13818=CARTESIAN_POINT('Ctrl Pts',(-0.588777006905475,-0.123392992551698,
1.79938991739155));
#13819=CARTESIAN_POINT('Ctrl Pts',(-0.580564309297537,-0.0793799999999999,
1.80203581326062));
#13820=CARTESIAN_POINT('Origin',(-0.962500000000001,-0.07938,1.66709890228504));
#13821=CARTESIAN_POINT('Origin',(0.,-0.07938,0.));
#13822=CARTESIAN_POINT('',(-1.60306435598592,-0.07938,1.00725997640701));
#13823=CARTESIAN_POINT('Origin',(0.,-0.07938,0.));
#13824=CARTESIAN_POINT('Origin',(-1.80890829501287,-0.07938,0.658388775901912));
#13825=CARTESIAN_POINT('Origin',(-1.80890829501287,0.,0.658388775901912));
#13826=CARTESIAN_POINT('',(-1.8754727744327,-0.07938,0.258823997855139));
#13827=CARTESIAN_POINT('Ctrl Pts',(-1.8754727744327,-0.07938,0.258823997855138));
#13828=CARTESIAN_POINT('Ctrl Pts',(-1.87429319564052,-0.123392992551698,
0.267371381128541));
#13829=CARTESIAN_POINT('Ctrl Pts',(-1.87207293588642,-0.166529565724165,
0.283268822605344));
#13830=CARTESIAN_POINT('Ctrl Pts',(-1.86551115062085,-0.237213819614884,
0.323392218961362));
#13831=CARTESIAN_POINT('Ctrl Pts',(-1.86166224891746,-0.266247928944116,
0.34532483272118));
#13832=CARTESIAN_POINT('Ctrl Pts',(-1.85170818356893,-0.317173992396757,
0.395237108747477));
#13833=CARTESIAN_POINT('Ctrl Pts',(-1.84558854251276,-0.339063173951852,
0.423216711561106));
#13834=CARTESIAN_POINT('Ctrl Pts',(-1.83135774191,-0.373566122196588,0.481006384765672));
#13835=CARTESIAN_POINT('Ctrl Pts',(-1.82255520314685,-0.388075792674377,
0.513732289895913));
#13836=CARTESIAN_POINT('Ctrl Pts',(-1.8021878073054,-0.407069005705619,
0.581160429138046));
#13837=CARTESIAN_POINT('Ctrl Pts',(-1.79059939410895,-0.411552957311693,
0.615855430396488));
#13838=CARTESIAN_POINT('Ctrl Pts',(-1.76754295572641,-0.411552957311693,
0.679202474225583));
#13839=CARTESIAN_POINT('Ctrl Pts',(-1.75411867833313,-0.407069005705619,
0.713229275562222));
#13840=CARTESIAN_POINT('Ctrl Pts',(-1.72637903628921,-0.388075792674378,
0.777974136626975));
#13841=CARTESIAN_POINT('Ctrl Pts',(-1.71208636586057,-0.373566122196588,
0.808701797248777));
#13842=CARTESIAN_POINT('Ctrl Pts',(-1.68584130567972,-0.339063173951852,
0.862118637580169));
#13843=CARTESIAN_POINT('Ctrl Pts',(-1.67254428069212,-0.317173992396757,
0.88748588628286));
#13844=CARTESIAN_POINT('Ctrl Pts',(-1.64808654453785,-0.266247928944116,
0.932119257848273));
#13845=CARTESIAN_POINT('Ctrl Pts',(-1.63693696192699,-0.237213819614884,
0.951394641067894));
#13846=CARTESIAN_POINT('Ctrl Pts',(-1.61617275903043,-0.166529565724165,
0.986348780151617));
#13847=CARTESIAN_POINT('Ctrl Pts',(-1.60765489827034,-0.123392992551698,
0.999954082314951));
#13848=CARTESIAN_POINT('Ctrl Pts',(-1.60306435598592,-0.07938,1.00725997640701));
#13849=CARTESIAN_POINT('Origin',(-1.80890829501287,-0.07938,0.658388775901912));
#13850=CARTESIAN_POINT('Origin',(0.,-0.07938,0.));
#13851=CARTESIAN_POINT('',(-1.893248,-0.0793799999999999,2.31856010319213E-16));
#13852=CARTESIAN_POINT('Origin',(0.,-0.07938,0.));
#13853=CARTESIAN_POINT('',(-1.8754727744327,-0.07938,-0.258823997855139));
#13854=CARTESIAN_POINT('Origin',(0.,-0.07938,0.));
#13855=CARTESIAN_POINT('Origin',(-1.80890829501287,-0.07938,-0.658388775901913));
#13856=CARTESIAN_POINT('Origin',(-1.80890829501287,0.,-0.658388775901913));
#13857=CARTESIAN_POINT('',(-1.60306435598592,-0.07938,-1.00725997640701));
#13858=CARTESIAN_POINT('Ctrl Pts',(-1.60306435598592,-0.07938,-1.00725997640701));
#13859=CARTESIAN_POINT('Ctrl Pts',(-1.60765489827034,-0.123392992551698,
-0.999954082314952));
#13860=CARTESIAN_POINT('Ctrl Pts',(-1.61617275903043,-0.166529565724166,
-0.986348780151617));
#13861=CARTESIAN_POINT('Ctrl Pts',(-1.63693696192699,-0.237213819614884,
-0.951394641067894));
#13862=CARTESIAN_POINT('Ctrl Pts',(-1.64808654453785,-0.266247928944116,
-0.932119257848273));
#13863=CARTESIAN_POINT('Ctrl Pts',(-1.67254428069212,-0.317173992396757,
-0.88748588628286));
#13864=CARTESIAN_POINT('Ctrl Pts',(-1.68584130567972,-0.339063173951852,
-0.862118637580169));
#13865=CARTESIAN_POINT('Ctrl Pts',(-1.71208636586057,-0.373566122196588,
-0.808701797248777));
#13866=CARTESIAN_POINT('Ctrl Pts',(-1.72637903628921,-0.388075792674377,
-0.777974136626975));
#13867=CARTESIAN_POINT('Ctrl Pts',(-1.75411867833313,-0.407069005705619,
-0.713229275562223));
#13868=CARTESIAN_POINT('Ctrl Pts',(-1.76754295572641,-0.411552957311693,
-0.679202474225584));
#13869=CARTESIAN_POINT('Ctrl Pts',(-1.79059939410895,-0.411552957311693,
-0.615855430396488));
#13870=CARTESIAN_POINT('Ctrl Pts',(-1.8021878073054,-0.407069005705619,
-0.581160429138047));
#13871=CARTESIAN_POINT('Ctrl Pts',(-1.82255520314685,-0.388075792674378,
-0.513732289895914));
#13872=CARTESIAN_POINT('Ctrl Pts',(-1.83135774191,-0.373566122196588,-0.481006384765673));
#13873=CARTESIAN_POINT('Ctrl Pts',(-1.84558854251276,-0.339063173951852,
-0.423216711561107));
#13874=CARTESIAN_POINT('Ctrl Pts',(-1.85170818356893,-0.317173992396757,
-0.395237108747477));
#13875=CARTESIAN_POINT('Ctrl Pts',(-1.86166224891746,-0.266247928944116,
-0.34532483272118));
#13876=CARTESIAN_POINT('Ctrl Pts',(-1.86551115062085,-0.237213819614884,
-0.323392218961362));
#13877=CARTESIAN_POINT('Ctrl Pts',(-1.87207293588642,-0.166529565724166,
-0.283268822605344));
#13878=CARTESIAN_POINT('Ctrl Pts',(-1.87429319564052,-0.123392992551698,
-0.267371381128542));
#13879=CARTESIAN_POINT('Ctrl Pts',(-1.8754727744327,-0.07938,-0.258823997855139));
#13880=CARTESIAN_POINT('Origin',(-1.80890829501287,-0.07938,-0.658388775901913));
#13881=CARTESIAN_POINT('Origin',(0.,-0.07938,0.));
#13882=CARTESIAN_POINT('',(-1.27032663816428,-0.07938,-1.40380134701254));
#13883=CARTESIAN_POINT('Origin',(0.,-0.07938,0.));
#13884=CARTESIAN_POINT('Origin',(-0.9625,-0.07938,-1.66709890228504));
#13885=CARTESIAN_POINT('Origin',(-0.9625,0.,-1.66709890228504));
#13886=CARTESIAN_POINT('',(-0.580564309297535,-0.07938,-1.80203581326062));
#13887=CARTESIAN_POINT('Ctrl Pts',(-0.580564309297535,-0.07938,-1.80203581326062));
#13888=CARTESIAN_POINT('Ctrl Pts',(-0.588777006905474,-0.123392992551698,
-1.79938991739155));
#13889=CARTESIAN_POINT('Ctrl Pts',(-0.60404738646464,-0.166529565724165,
-1.79444282663));
#13890=CARTESIAN_POINT('Ctrl Pts',(-0.642421776219619,-0.237213819614884,
-1.78101337496783));
#13891=CARTESIAN_POINT('Ctrl Pts',(-0.663352829527298,-0.266247928944116,
-1.77341438831889));
#13892=CARTESIAN_POINT('Ctrl Pts',(-0.71077832062033,-0.317173992396757,
-1.75494437181449));
#13893=CARTESIAN_POINT('Ctrl Pts',(-0.737270185880015,-0.339063173951852,
-1.74405909481629));
#13894=CARTESIAN_POINT('Ctrl Pts',(-0.791710751504504,-0.373566122196588,
-1.72000942061118));
#13895=CARTESIAN_POINT('Ctrl Pts',(-0.822410931786042,-0.388075792674378,
-1.70565781840267));
#13896=CARTESIAN_POINT('Ctrl Pts',(-0.885277924911194,-0.407069005705619,
-1.67389107556648));
#13897=CARTESIAN_POINT('Ctrl Pts',(-0.917433524307661,-0.411552957311693,
-1.65645399266283));
#13898=CARTESIAN_POINT('Ctrl Pts',(-0.975814475692338,-0.411552957311693,
-1.62274773466534));
#13899=CARTESIAN_POINT('Ctrl Pts',(-1.00699323215303,-0.407069005705619,
-1.60361871016591));
#13900=CARTESIAN_POINT('Ctrl Pts',(-1.06593753500724,-0.388075792674378,
-1.56505766847808));
#13901=CARTESIAN_POINT('Ctrl Pts',(-1.09371647724559,-0.373566122196588,
-1.54564633355776));
#13902=CARTESIAN_POINT('Ctrl Pts',(-1.14176438887219,-0.339063173951852,
-1.51052425783311));
#13903=CARTESIAN_POINT('Ctrl Pts',(-1.1644372479097,-0.317173992396757,
-1.49302426802369));
#13904=CARTESIAN_POINT('Ctrl Pts',(-1.20414549695735,-0.266247928944116,
-1.46118759620237));
#13905=CARTESIAN_POINT('Ctrl Pts',(-1.22119193909219,-0.237213819614884,
-1.44686026563443));
#13906=CARTESIAN_POINT('Ctrl Pts',(-1.25200938026802,-0.166529565724166,
-1.42034179508298));
#13907=CARTESIAN_POINT('Ctrl Pts',(-1.26392887632193,-0.123392992551698,
-1.40959080384008));
#13908=CARTESIAN_POINT('Ctrl Pts',(-1.27032663816428,-0.07938,-1.40380134701254));
#13909=CARTESIAN_POINT('Origin',(-0.9625,-0.07938,-1.66709890228504));
#13910=CARTESIAN_POINT('Origin',(0.,-0.07938,0.));
#13911=CARTESIAN_POINT('',(-0.0707805497908242,-0.07938,-1.89192444438865));
#13912=CARTESIAN_POINT('Origin',(0.,-0.07938,0.));
#13913=CARTESIAN_POINT('Origin',(0.334272742008841,-0.07938,-1.8957549245485));
#13914=CARTESIAN_POINT('Origin',(0.334272742008841,0.,-1.8957549245485));
#13915=CARTESIAN_POINT('',(0.71358822996475,-0.07938,-1.75361906569237));
#13916=CARTESIAN_POINT('Ctrl Pts',(0.71358822996475,-0.07938,-1.75361906569237));
#13917=CARTESIAN_POINT('Ctrl Pts',(0.705596189518014,-0.123392992551698,
-1.75687121212928));
#13918=CARTESIAN_POINT('Ctrl Pts',(0.690718471466876,-0.166529565724166,
-1.76289713151763));
#13919=CARTESIAN_POINT('Ctrl Pts',(0.652689698303666,-0.237213819614884,
-1.77727615696148));
#13920=CARTESIAN_POINT('Ctrl Pts',(0.631771046764578,-0.266247928944116,
-1.78490921718958));
#13921=CARTESIAN_POINT('Ctrl Pts',(0.583568715090837,-0.317173992396757,
-1.80124488173997));
#13922=CARTESIAN_POINT('Ctrl Pts',(0.556277847738351,-0.339063173951852,
-1.8099349185301));
#13923=CARTESIAN_POINT('Ctrl Pts',(0.499115122365417,-0.373566122196588,
-1.8265055202942));
#13924=CARTESIAN_POINT('Ctrl Pts',(0.466372387779211,-0.388075792674378,
-1.83524525067263));
#13925=CARTESIAN_POINT('Ctrl Pts',(0.397794208344886,-0.407069005705619,
-1.85132063808607));
#13926=CARTESIAN_POINT('Ctrl Pts',(0.361953249272519,-0.411552957311693,
-1.85863227849762));
#13927=CARTESIAN_POINT('Ctrl Pts',(0.295564880870602,-0.411552957311693,
-1.87033833905209));
#13928=CARTESIAN_POINT('Ctrl Pts',(0.259384667806906,-0.407069005705619,
-1.87572597447038));
#13929=CARTESIAN_POINT('Ctrl Pts',(0.189444152338379,-0.388075792674377,
-1.88407517030084));
#13930=CARTESIAN_POINT('Ctrl Pts',(0.155686882426711,-0.373566122196588,
-1.88706118493262));
#13931=CARTESIAN_POINT('Ctrl Pts',(0.096304011619402,-0.339063173951852,
-1.89104071625784));
#13932=CARTESIAN_POINT('Ctrl Pts',(0.0676868173249583,-0.317173992396757,
-1.89220877917518));
#13933=CARTESIAN_POINT('Ctrl Pts',(0.0168043156156251,-0.266247928944116,
-1.89334444412923));
#13934=CARTESIAN_POINT('Ctrl Pts',(-0.00546344722567807,-0.237213819614884,
-1.89332631395644));
#13935=CARTESIAN_POINT('Ctrl Pts',(-0.0461167210878748,-0.166529565724165,
-1.89282105630055));
#13936=CARTESIAN_POINT('Ctrl Pts',(-0.0621581887675344,-0.123392992551698,
-1.89224702357808));
#13937=CARTESIAN_POINT('Ctrl Pts',(-0.0707805497908242,-0.07938,-1.89192444438865));
#13938=CARTESIAN_POINT('Origin',(0.334272742008841,-0.07938,-1.8957549245485));
#13939=CARTESIAN_POINT('Origin',(0.,-0.07938,0.));
#13940=CARTESIAN_POINT('',(1.16188454446795,-0.07938,-1.49479506783723));
#13941=CARTESIAN_POINT('Origin',(0.,-0.07938,0.));
#13942=CARTESIAN_POINT('Origin',(1.47463555300403,-0.07938,-1.23736614864659));
#13943=CARTESIAN_POINT('Origin',(1.47463555300403,0.,-1.23736614864659));
#13944=CARTESIAN_POINT('',(1.67384490577674,-0.07938,-0.884664467981643));
#13945=CARTESIAN_POINT('Ctrl Pts',(1.67384490577674,-0.07938,-0.884664467981643));
#13946=CARTESIAN_POINT('Ctrl Pts',(1.66981308703787,-0.123392992551698,
-0.892292941263125));
#13947=CARTESIAN_POINT('Ctrl Pts',(1.66228948011831,-0.166529565724165,
-0.906472276148934));
#13948=CARTESIAN_POINT('Ctrl Pts',(1.64240040915267,-0.237213819614884,
-0.941931672888549));
#13949=CARTESIAN_POINT('Ctrl Pts',(1.63128222892223,-0.266247928944116,
-0.961225186280958));
#13950=CARTESIAN_POINT('Ctrl Pts',(1.60485746336717,-0.317173992396757,
-1.00472289289232));
#13951=CARTESIAN_POINT('Ctrl Pts',(1.58953729406031,-0.339063173951852,
-1.02892207867768));
#13952=CARTESIAN_POINT('Ctrl Pts',(1.55639948343386,-0.373566122196588,
-1.07835938768384));
#13953=CARTESIAN_POINT('Ctrl Pts',(1.53693488395083,-0.388075792674377,
-1.10610103367386));
#13954=CARTESIAN_POINT('Ctrl Pts',(1.49473401052622,-0.407069005705619,
-1.16249669890816));
#13955=CARTESIAN_POINT('Ctrl Pts',(1.4719780748558,-0.411552957311693,-1.19113586482651));
#13956=CARTESIAN_POINT('Ctrl Pts',(1.42864614483643,-0.411552957311693,
-1.24277684810113));
#13957=CARTESIAN_POINT('Ctrl Pts',(1.40439359896051,-0.407069005705619,
-1.27016020894803));
#13958=CARTESIAN_POINT('Ctrl Pts',(1.35618281536764,-0.388075792674378,
-1.32151296077672));
#13959=CARTESIAN_POINT('Ctrl Pts',(1.33224261954459,-0.373566122196588,
-1.34549913552853));
#13960=CARTESIAN_POINT('Ctrl Pts',(1.28931069477441,-0.339063173951852,
-1.38671820696899));
#13961=CARTESIAN_POINT('Ctrl Pts',(1.26813946847809,-0.317173992396757,
-1.40600777299249));
#13962=CARTESIAN_POINT('Ctrl Pts',(1.22989120215289,-0.266247928944116,
-1.4395843844684));
#13963=CARTESIAN_POINT('Ctrl Pts',(1.21282145231718,-0.237213819614884,
-1.45388393800011));
#13964=CARTESIAN_POINT('Ctrl Pts',(1.18135446441955,-0.166529565724166,
-1.47962830891229));
#13965=CARTESIAN_POINT('Ctrl Pts',(1.16869700612251,-0.123392992551698,
-1.48949983100074));
#13966=CARTESIAN_POINT('Ctrl Pts',(1.16188454446795,-0.0793799999999999,
-1.49479506783723));
#13967=CARTESIAN_POINT('Origin',(1.47463555300403,-0.07938,-1.23736614864659));
#13968=CARTESIAN_POINT('Origin',(0.,-0.27783,0.));
#13969=CARTESIAN_POINT('',(-1.893248,-0.47628,2.31856010319213E-16));
#13970=CARTESIAN_POINT('Origin',(0.,-0.47628,0.));
#13971=CARTESIAN_POINT('',(-1.893248,-0.27783,2.31856010319213E-16));
#13972=CARTESIAN_POINT('',(1.85089094746182,-0.07938,0.39823446624808));
#13973=CARTESIAN_POINT('Origin',(0.,-0.07938,0.));
#13974=CARTESIAN_POINT('',(1.85089094746182,-0.07938,-0.39823446624808));
#13975=CARTESIAN_POINT('Ctrl Pts',(1.85089094746182,-0.07938,0.39823446624808));
#13976=CARTESIAN_POINT('Ctrl Pts',(1.8527058832274,-0.123392992551698,0.38979911355147));
#13977=CARTESIAN_POINT('Ctrl Pts',(1.85605676673266,-0.166529565724166,
0.374101031547026));
#13978=CARTESIAN_POINT('Ctrl Pts',(1.86361371531181,-0.237213819614884,
0.334153109333404));
#13979=CARTESIAN_POINT('Ctrl Pts',(1.86749832648465,-0.266247928944116,
0.312226792116516));
#13980=CARTESIAN_POINT('Ctrl Pts',(1.87521556853004,-0.317173992396757,
0.261920103790797));
#13981=CARTESIAN_POINT('Ctrl Pts',(1.87903457475221,-0.339063173951852,
0.233534836983177));
#13982=CARTESIAN_POINT('Ctrl Pts',(1.88542722875009,-0.373566122196588,
0.174363087053423));
#13983=CARTESIAN_POINT('Ctrl Pts',(1.88834846679328,-0.388075792674378,
0.140600149924591));
#13984=CARTESIAN_POINT('Ctrl Pts',(1.89227115706422,-0.407069005705619,
0.0702723654005715));
#13985=CARTESIAN_POINT('Ctrl Pts',(1.893248,-0.411552957311693,0.0337062579974903));
#13986=CARTESIAN_POINT('Ctrl Pts',(1.893248,-0.411552957311693,-0.0337062579974903));
#13987=CARTESIAN_POINT('Ctrl Pts',(1.89227115706422,-0.407069005705619,
-0.0702723654005715));
#13988=CARTESIAN_POINT('Ctrl Pts',(1.88834846679328,-0.388075792674378,
-0.140600149924591));
#13989=CARTESIAN_POINT('Ctrl Pts',(1.88542722875009,-0.373566122196588,
-0.174363087053422));
#13990=CARTESIAN_POINT('Ctrl Pts',(1.87903457475221,-0.339063173951852,
-0.233534836983177));
#13991=CARTESIAN_POINT('Ctrl Pts',(1.87521556853004,-0.317173992396757,
-0.261920103790797));
#13992=CARTESIAN_POINT('Ctrl Pts',(1.86749832648465,-0.266247928944116,
-0.312226792116516));
#13993=CARTESIAN_POINT('Ctrl Pts',(1.86361371531181,-0.237213819614884,
-0.334153109333404));
#13994=CARTESIAN_POINT('Ctrl Pts',(1.85605676673266,-0.166529565724166,
-0.374101031547026));
#13995=CARTESIAN_POINT('Ctrl Pts',(1.8527058832274,-0.123392992551698,-0.38979911355147));
#13996=CARTESIAN_POINT('Ctrl Pts',(1.85089094746182,-0.07938,-0.39823446624808));
#13997=CARTESIAN_POINT('Origin',(0.,-0.07938,0.));
#13998=CARTESIAN_POINT('Origin',(0.,-0.07938,0.));
#13999=CARTESIAN_POINT('Origin',(1.925,-0.07938,0.));
#14000=CARTESIAN_POINT('Origin',(1.925,0.,0.));
#14001=CARTESIAN_POINT('Origin',(1.925,-0.07938,0.));
#14002=CARTESIAN_POINT('Origin',(0.,-0.47628,0.));
#14003=CARTESIAN_POINT('Origin',(0.,-0.07938,0.));
#16154=UNCERTAINTY_MEASURE_WITH_UNIT(LENGTH_MEASURE(0.001),#16282,
'DISTANCE_ACCURACY_VALUE',
'Maximum model space distance between geometric entities at asserted c
onnectivities');
#16212=UNCERTAINTY_MEASURE_WITH_UNIT(LENGTH_MEASURE(0.001),#16282,
'DISTANCE_ACCURACY_VALUE',
'Maximum model space distance between geometric entities at asserted c
onnectivities');
#16223=(
GEOMETRIC_REPRESENTATION_CONTEXT(3)
GLOBAL_UNCERTAINTY_ASSIGNED_CONTEXT((#16154))
GLOBAL_UNIT_ASSIGNED_CONTEXT((#16282,#16284,#16285))
REPRESENTATION_CONTEXT('','3D')
);
#16281=(
GEOMETRIC_REPRESENTATION_CONTEXT(3)
GLOBAL_UNCERTAINTY_ASSIGNED_CONTEXT((#16212))
GLOBAL_UNIT_ASSIGNED_CONTEXT((#16282,#16284,#16285))
REPRESENTATION_CONTEXT('','3D')
);
#16282=(
LENGTH_UNIT()
NAMED_UNIT(*)
SI_UNIT(.CENTI.,.METRE.)
);
#16284=(
NAMED_UNIT(*)
PLANE_ANGLE_UNIT()
SI_UNIT($,.RADIAN.)
);
#16285=(
NAMED_UNIT(*)
SI_UNIT($,.STERADIAN.)
SOLID_ANGLE_UNIT()
);
#16296=SHAPE_DEFINITION_REPRESENTATION(#16364,#16529);
#16364=PRODUCT_DEFINITION_SHAPE('',$,#16598);
#16529=SHAPE_REPRESENTATION('',(#9290),#16223);
#16587=PRODUCT_DEFINITION_CONTEXT('part definition',#16793,'design');
#16598=PRODUCT_DEFINITION('Cage','Cage',#16666,#16587);
#16666=PRODUCT_DEFINITION_FORMATION('',$,#16805);
#16793=APPLICATION_CONTEXT(
'Core Data for Automotive Mechanical Design Process');
#16794=PRODUCT_CONTEXT('part definition',#16793,'mechanical');
#16805=PRODUCT('Cage','Cage','Cage',(#16794));
#16926=COLOUR_RGB('Grey',0.48,0.52,0.57);
#16927=FILL_AREA_STYLE_COLOUR('',#16926);
#16928=FILL_AREA_STYLE('',(#16927));
#16929=SURFACE_STYLE_FILL_AREA(#16928);
#16930=SURFACE_SIDE_STYLE('',(#16929));
#16931=SURFACE_STYLE_USAGE(.BOTH.,#16930);
#16932=PRESENTATION_STYLE_ASSIGNMENT((#16931));
ENDSEC;
END-ISO-10303-21;
